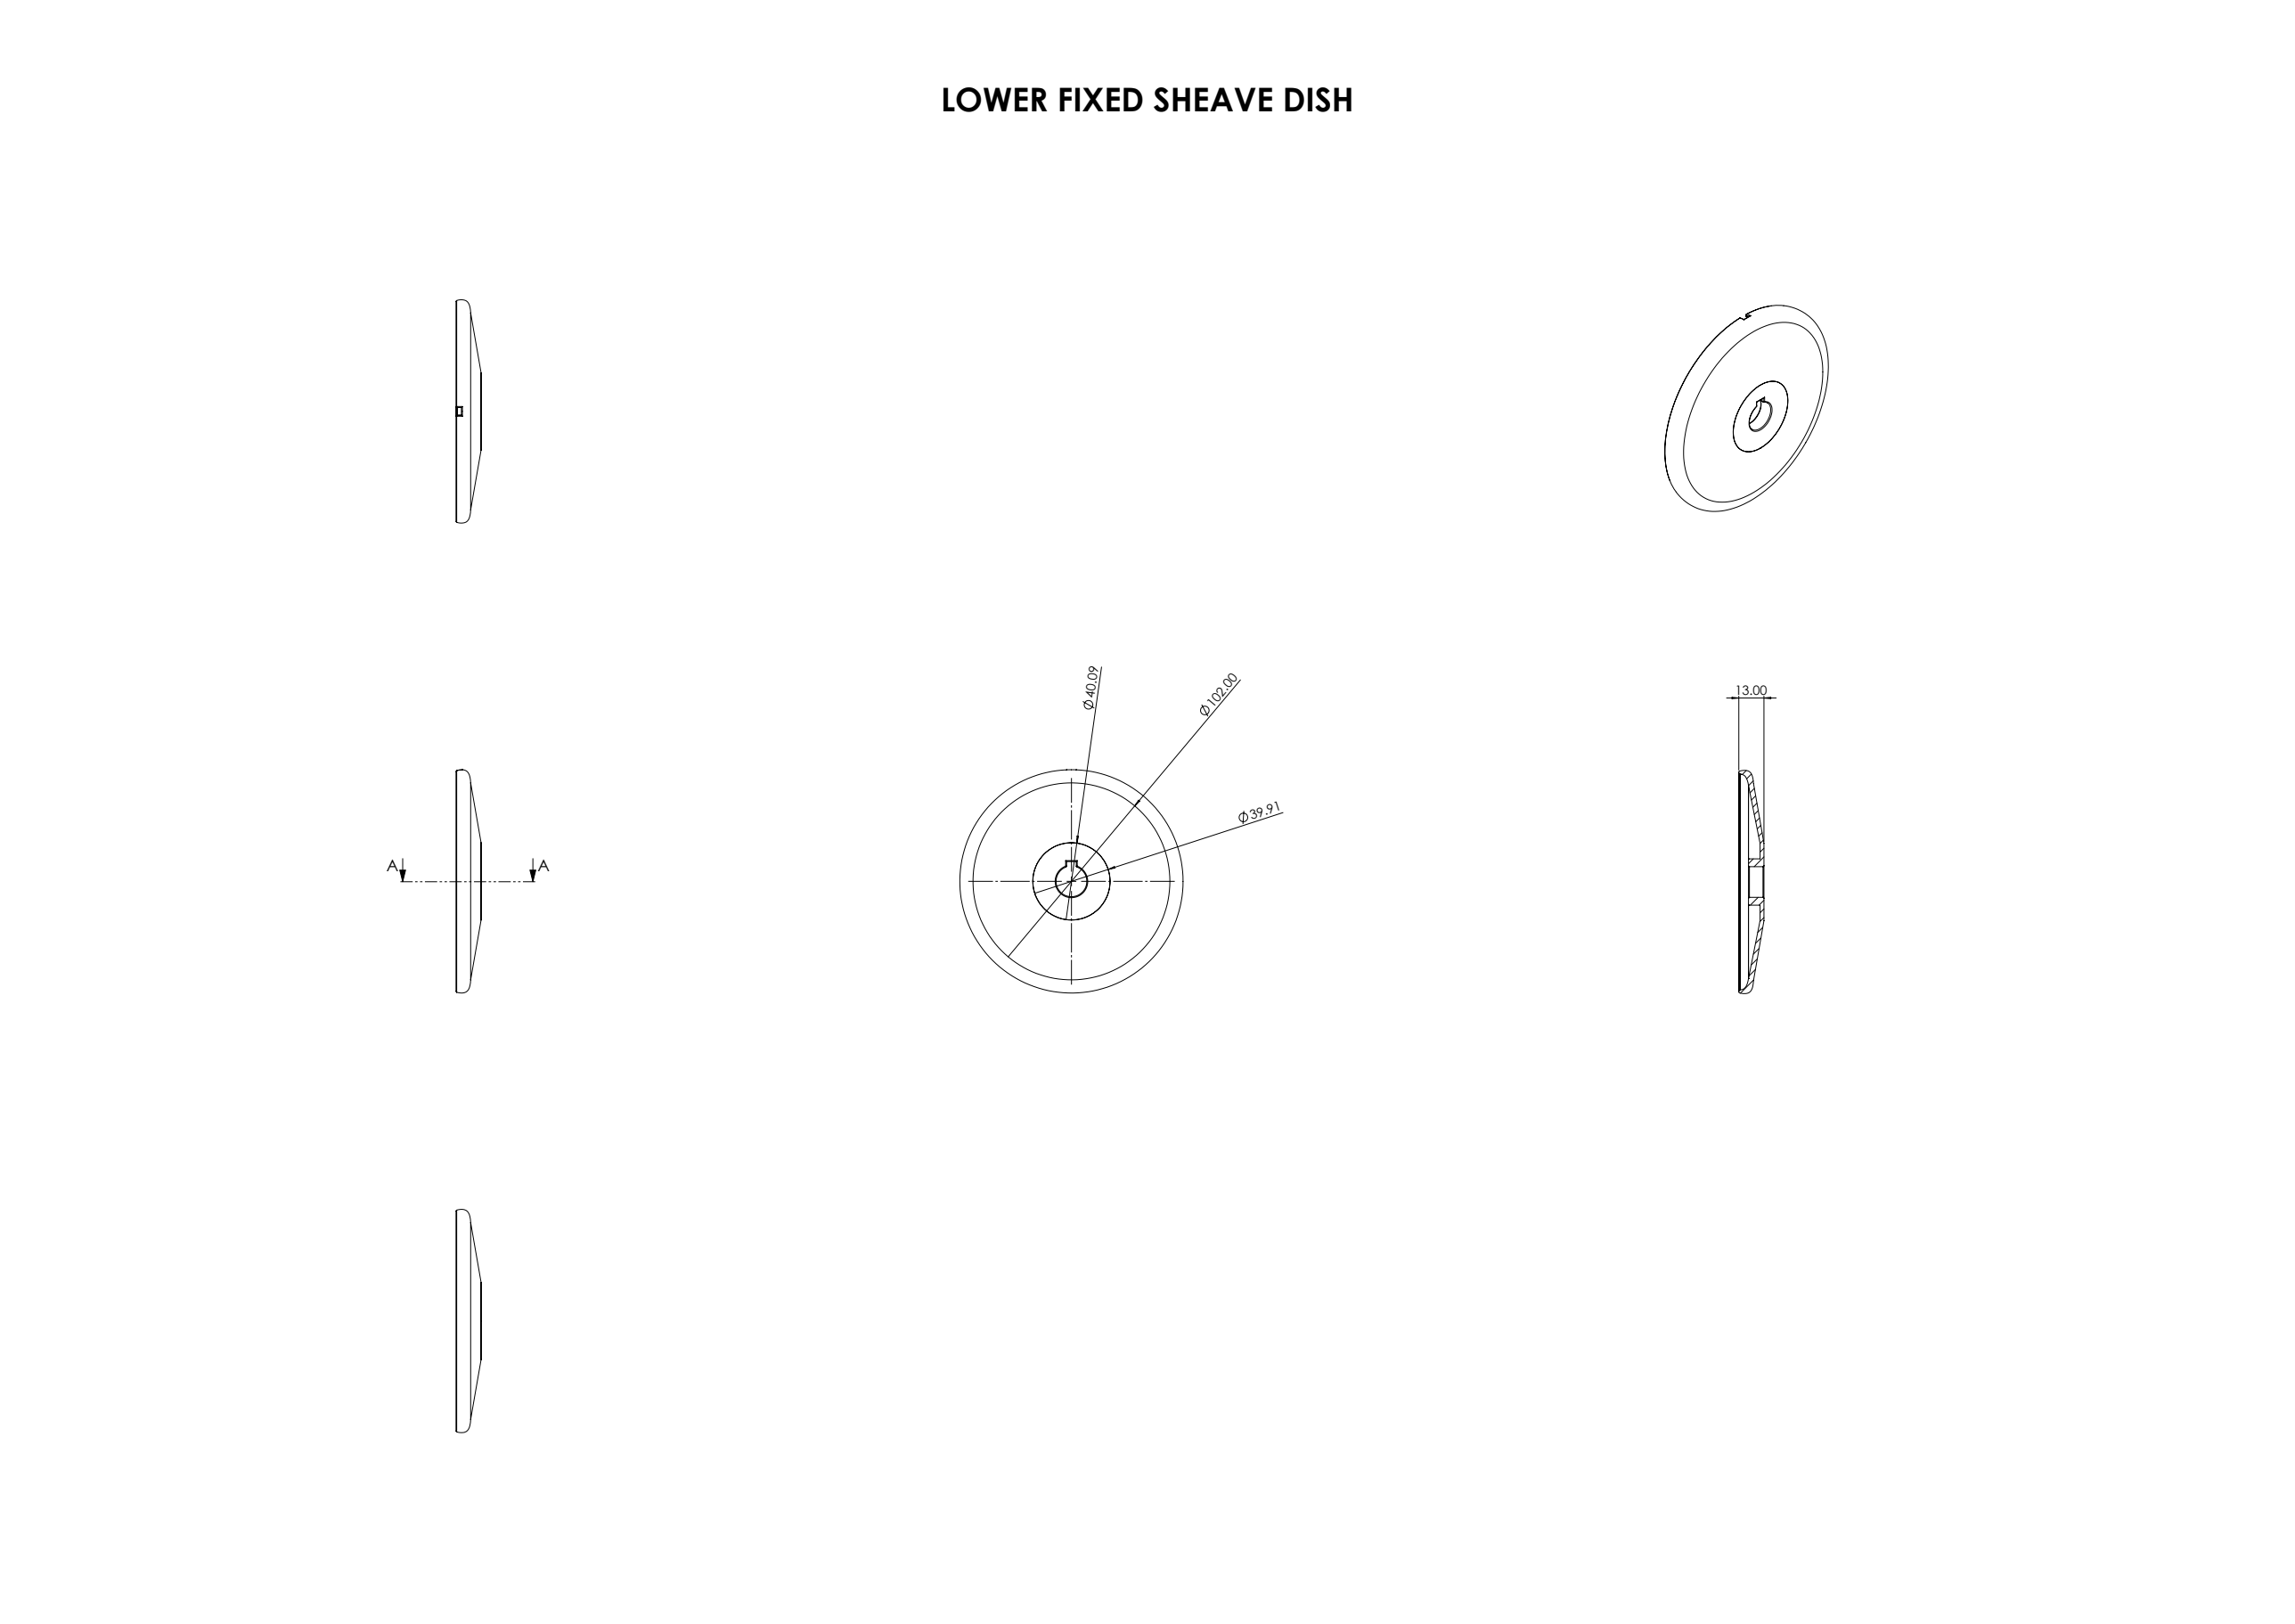
ISO-10303-21;
HEADER;
/* Generated by software containing ST-Developer
 * from STEP Tools, Inc. (www.steptools.com) 
 */

FILE_DESCRIPTION(
/* description */ (''),
/* implementation_level */ '2;1');

FILE_NAME(
/* name */ '04_Lower_Fixed_Sheave_Dish.step',
/* time_stamp */ '2026-10-24T13:41:11-07:00',
/* author */ (''),
/* organization */ (''),
/* preprocessor_version */ 'ST-DEVELOPER v20.2',
/* originating_system */ 'Autodesk Translation Framework v15.15.0.0',
/* authorisation */ '');

FILE_SCHEMA (('AUTOMOTIVE_DESIGN { 1 0 10303 214 3 1 1 }'));
ENDSEC;

DATA;
#10=MECHANICAL_DESIGN_GEOMETRIC_PRESENTATION_REPRESENTATION('',(#124),#12813);
#63=ELLIPSE('',#4739,0.707106781186547,0.5);
#64=ELLIPSE('',#4740,0.707106781186547,0.5);
#65=ELLIPSE('',#4754,0.707106781186549,0.5);
#66=ELLIPSE('',#4755,0.707106781186547,0.5);
#67=SPHERICAL_SURFACE('',#4710,0.5);
#68=SPHERICAL_SURFACE('',#4712,0.5);
#69=SPHERICAL_SURFACE('',#4720,0.5);
#70=SPHERICAL_SURFACE('',#4723,0.5);
#71=SPHERICAL_SURFACE('',#4743,0.5);
#72=SPHERICAL_SURFACE('',#4756,0.5);
#73=SPHERICAL_SURFACE('',#4773,0.5);
#74=SPHERICAL_SURFACE('',#4779,0.5);
#75=SPHERICAL_SURFACE('',#4788,0.5);
#76=SPHERICAL_SURFACE('',#4790,0.5);
#89=CONICAL_SURFACE('',#4727,35.,1.37340076694502);
#90=CONICAL_SURFACE('',#4770,35.5,1.39833325526807);
#91=CONICAL_SURFACE('',#4795,56.05,0.694738276196701);
#104=SHAPE_REPRESENTATION_RELATIONSHIP('SRR','None',#12857,#114);
#114=ADVANCED_BREP_SHAPE_REPRESENTATION('',(#134),#12806);
#124=STYLED_ITEM('',(#12967),#134);
#134=MANIFOLD_SOLID_BREP('Body1',#4387);
#153=FACE_BOUND('',#738,.T.);
#154=FACE_BOUND('',#753,.T.);
#155=FACE_BOUND('',#774,.T.);
#196=PLANE('',#4717);
#197=PLANE('',#4725);
#198=PLANE('',#4734);
#199=PLANE('',#4751);
#200=PLANE('',#4752);
#201=PLANE('',#4769);
#202=PLANE('',#4781);
#203=PLANE('',#4792);
#204=PLANE('',#4793);
#205=PLANE('',#4794);
#272=TOROIDAL_SURFACE('',#4705,56.5341874729922,0.5);
#273=TOROIDAL_SURFACE('',#4729,11.5,0.5);
#274=TOROIDAL_SURFACE('',#4746,8.45,0.5);
#275=TOROIDAL_SURFACE('',#4760,8.45,0.5);
#276=TOROIDAL_SURFACE('',#4764,19.9567770454363,0.5);
#292=(
BOUNDED_CURVE()
B_SPLINE_CURVE(5,(#10926,#10927,#10928,#10929,#10930,#10931,#10932,#10933,
#10934,#10935,#10936,#10937,#10938,#10939,#10940),.UNSPECIFIED.,.F.,.F.)
B_SPLINE_CURVE_WITH_KNOTS((6,1,1,1,1,1,1,1,1,1,6),(0.000900413620571326,
0.0666666666666667,0.133333333333333,0.2,0.266666666666667,0.333333333333333,
0.4,0.466666666666667,0.533333333333333,0.6,0.62572757688512),
 .UNSPECIFIED.)
CURVE()
GEOMETRIC_REPRESENTATION_ITEM()
RATIONAL_B_SPLINE_CURVE((1.,1.,1.,1.,1.,1.,1.,1.,1.,1.,1.,1.,1.,1.,1.))
REPRESENTATION_ITEM('')
);
#293=(
BOUNDED_CURVE()
B_SPLINE_CURVE(5,(#11656,#11657,#11658,#11659,#11660,#11661,#11662,#11663,
#11664,#11665,#11666,#11667,#11668,#11669,#11670,#11671,#11672,#11673,#11674),
 .UNSPECIFIED.,.F.,.F.)
B_SPLINE_CURVE_WITH_KNOTS((6,1,1,1,1,1,1,1,1,1,1,1,1,1,6),(0.323025444096601,
0.35,0.4,0.45,0.5,0.55,0.6,0.65,0.7,0.75,0.8,0.85,0.9,0.95,1.),
 .UNSPECIFIED.)
CURVE()
GEOMETRIC_REPRESENTATION_ITEM()
RATIONAL_B_SPLINE_CURVE((1.,1.,1.,1.,1.,1.,1.,1.,1.,1.,1.,1.,1.,1.,1.,1.,
1.,1.,1.))
REPRESENTATION_ITEM('')
);
#296=(
BOUNDED_SURFACE()
B_SPLINE_SURFACE(5,2,((#10735,#10736,#10737,#10738,#10739,#10740,#10741,
#10742,#10743),(#10744,#10745,#10746,#10747,#10748,#10749,#10750,#10751,
#10752),(#10753,#10754,#10755,#10756,#10757,#10758,#10759,#10760,#10761),
(#10762,#10763,#10764,#10765,#10766,#10767,#10768,#10769,#10770),(#10771,
#10772,#10773,#10774,#10775,#10776,#10777,#10778,#10779),(#10780,#10781,
#10782,#10783,#10784,#10785,#10786,#10787,#10788),(#10789,#10790,#10791,
#10792,#10793,#10794,#10795,#10796,#10797),(#10798,#10799,#10800,#10801,
#10802,#10803,#10804,#10805,#10806),(#10807,#10808,#10809,#10810,#10811,
#10812,#10813,#10814,#10815),(#10816,#10817,#10818,#10819,#10820,#10821,
#10822,#10823,#10824),(#10825,#10826,#10827,#10828,#10829,#10830,#10831,
#10832,#10833),(#10834,#10835,#10836,#10837,#10838,#10839,#10840,#10841,
#10842),(#10843,#10844,#10845,#10846,#10847,#10848,#10849,#10850,#10851),
(#10852,#10853,#10854,#10855,#10856,#10857,#10858,#10859,#10860),(#10861,
#10862,#10863,#10864,#10865,#10866,#10867,#10868,#10869),(#10870,#10871,
#10872,#10873,#10874,#10875,#10876,#10877,#10878),(#10879,#10880,#10881,
#10882,#10883,#10884,#10885,#10886,#10887),(#10888,#10889,#10890,#10891,
#10892,#10893,#10894,#10895,#10896),(#10897,#10898,#10899,#10900,#10901,
#10902,#10903,#10904,#10905),(#10906,#10907,#10908,#10909,#10910,#10911,
#10912,#10913,#10914)),.UNSPECIFIED.,.F.,.T.,.F.)
B_SPLINE_SURFACE_WITH_KNOTS((6,1,1,1,1,1,1,1,1,1,1,1,1,1,1,6),(3,2,2,2,
3),(-1.,-0.933333333333333,-0.866666666666667,-0.8,-0.733333333333333,-0.666666666666667,
-0.6,-0.533333333333333,-0.466666666666667,-0.4,-0.333333333333333,-0.266666666666667,
-0.2,-0.133333333333333,-0.0666666666666667,0.),(0.,1.5707963267949,3.14159265358979,
4.71238898038469,6.28318530717959),.UNSPECIFIED.)
GEOMETRIC_REPRESENTATION_ITEM()
RATIONAL_B_SPLINE_SURFACE(((1.,0.707106781186548,1.,0.707106781186548,1.,
0.707106781186548,1.,0.707106781186548,1.),(1.,0.707106781186548,1.,0.707106781186548,
1.,0.707106781186548,1.,0.707106781186548,1.),(1.,0.707106781186548,1.,
0.707106781186548,1.,0.707106781186548,1.,0.707106781186548,1.),(1.,0.707106781186548,
1.,0.707106781186548,1.,0.707106781186548,1.,0.707106781186548,1.),(1.,
0.707106781186548,1.,0.707106781186548,1.,0.707106781186548,1.,0.707106781186548,
1.),(1.,0.707106781186548,1.,0.707106781186548,1.,0.707106781186548,1.,
0.707106781186548,1.),(1.,0.707106781186548,1.,0.707106781186548,1.,0.707106781186548,
1.,0.707106781186548,1.),(1.,0.707106781186548,1.,0.707106781186548,1.,
0.707106781186548,1.,0.707106781186548,1.),(1.,0.707106781186548,1.,0.707106781186548,
1.,0.707106781186548,1.,0.707106781186548,1.),(1.,0.707106781186548,1.,
0.707106781186548,1.,0.707106781186548,1.,0.707106781186548,1.),(1.,0.707106781186548,
1.,0.707106781186548,1.,0.707106781186548,1.,0.707106781186548,1.),(1.,
0.707106781186548,1.,0.707106781186548,1.,0.707106781186548,1.,0.707106781186548,
1.),(1.,0.707106781186548,1.,0.707106781186548,1.,0.707106781186548,1.,
0.707106781186548,1.),(1.,0.707106781186548,1.,0.707106781186548,1.,0.707106781186548,
1.,0.707106781186548,1.),(1.,0.707106781186548,1.,0.707106781186548,1.,
0.707106781186548,1.,0.707106781186548,1.),(1.,0.707106781186548,1.,0.707106781186548,
1.,0.707106781186548,1.,0.707106781186548,1.),(1.,0.707106781186548,1.,
0.707106781186548,1.,0.707106781186548,1.,0.707106781186548,1.),(1.,0.707106781186548,
1.,0.707106781186548,1.,0.707106781186548,1.,0.707106781186548,1.),(1.,
0.707106781186548,1.,0.707106781186548,1.,0.707106781186548,1.,0.707106781186548,
1.),(1.,0.707106781186548,1.,0.707106781186548,1.,0.707106781186548,1.,
0.707106781186548,1.)))
REPRESENTATION_ITEM('')
SURFACE()
);
#297=(
BOUNDED_SURFACE()
B_SPLINE_SURFACE(5,2,((#11421,#11422,#11423,#11424,#11425,#11426,#11427,
#11428,#11429),(#11430,#11431,#11432,#11433,#11434,#11435,#11436,#11437,
#11438),(#11439,#11440,#11441,#11442,#11443,#11444,#11445,#11446,#11447),
(#11448,#11449,#11450,#11451,#11452,#11453,#11454,#11455,#11456),(#11457,
#11458,#11459,#11460,#11461,#11462,#11463,#11464,#11465),(#11466,#11467,
#11468,#11469,#11470,#11471,#11472,#11473,#11474),(#11475,#11476,#11477,
#11478,#11479,#11480,#11481,#11482,#11483),(#11484,#11485,#11486,#11487,
#11488,#11489,#11490,#11491,#11492),(#11493,#11494,#11495,#11496,#11497,
#11498,#11499,#11500,#11501),(#11502,#11503,#11504,#11505,#11506,#11507,
#11508,#11509,#11510),(#11511,#11512,#11513,#11514,#11515,#11516,#11517,
#11518,#11519),(#11520,#11521,#11522,#11523,#11524,#11525,#11526,#11527,
#11528),(#11529,#11530,#11531,#11532,#11533,#11534,#11535,#11536,#11537),
(#11538,#11539,#11540,#11541,#11542,#11543,#11544,#11545,#11546),(#11547,
#11548,#11549,#11550,#11551,#11552,#11553,#11554,#11555),(#11556,#11557,
#11558,#11559,#11560,#11561,#11562,#11563,#11564),(#11565,#11566,#11567,
#11568,#11569,#11570,#11571,#11572,#11573),(#11574,#11575,#11576,#11577,
#11578,#11579,#11580,#11581,#11582),(#11583,#11584,#11585,#11586,#11587,
#11588,#11589,#11590,#11591),(#11592,#11593,#11594,#11595,#11596,#11597,
#11598,#11599,#11600),(#11601,#11602,#11603,#11604,#11605,#11606,#11607,
#11608,#11609),(#11610,#11611,#11612,#11613,#11614,#11615,#11616,#11617,
#11618),(#11619,#11620,#11621,#11622,#11623,#11624,#11625,#11626,#11627),
(#11628,#11629,#11630,#11631,#11632,#11633,#11634,#11635,#11636),(#11637,
#11638,#11639,#11640,#11641,#11642,#11643,#11644,#11645)),.UNSPECIFIED.,
 .F.,.T.,.F.)
B_SPLINE_SURFACE_WITH_KNOTS((6,1,1,1,1,1,1,1,1,1,1,1,1,1,1,1,1,1,1,1,6),
(3,2,2,2,3),(-1.,-0.95,-0.9,-0.85,-0.8,-0.75,-0.7,-0.65,-0.6,-0.55,-0.5,
-0.45,-0.4,-0.35,-0.3,-0.25,-0.2,-0.15,-0.1,-0.05,0.),(0.,1.5707963267949,
3.14159265358979,4.71238898038469,6.28318530717959),.UNSPECIFIED.)
GEOMETRIC_REPRESENTATION_ITEM()
RATIONAL_B_SPLINE_SURFACE(((1.,0.707106781186548,1.,0.707106781186548,1.,
0.707106781186548,1.,0.707106781186548,1.),(1.,0.707106781186548,1.,0.707106781186548,
1.,0.707106781186548,1.,0.707106781186548,1.),(1.,0.707106781186548,1.,
0.707106781186548,1.,0.707106781186548,1.,0.707106781186548,1.),(1.,0.707106781186548,
1.,0.707106781186548,1.,0.707106781186548,1.,0.707106781186548,1.),(1.,
0.707106781186548,1.,0.707106781186548,1.,0.707106781186548,1.,0.707106781186548,
1.),(1.,0.707106781186548,1.,0.707106781186548,1.,0.707106781186548,1.,
0.707106781186548,1.),(1.,0.707106781186548,1.,0.707106781186548,1.,0.707106781186548,
1.,0.707106781186548,1.),(1.,0.707106781186548,1.,0.707106781186548,1.,
0.707106781186548,1.,0.707106781186548,1.),(1.,0.707106781186548,1.,0.707106781186548,
1.,0.707106781186548,1.,0.707106781186548,1.),(1.,0.707106781186548,1.,
0.707106781186548,1.,0.707106781186548,1.,0.707106781186548,1.),(1.,0.707106781186548,
1.,0.707106781186548,1.,0.707106781186548,1.,0.707106781186548,1.),(1.,
0.707106781186548,1.,0.707106781186548,1.,0.707106781186548,1.,0.707106781186548,
1.),(1.,0.707106781186548,1.,0.707106781186548,1.,0.707106781186548,1.,
0.707106781186548,1.),(1.,0.707106781186548,1.,0.707106781186548,1.,0.707106781186548,
1.,0.707106781186548,1.),(1.,0.707106781186548,1.,0.707106781186548,1.,
0.707106781186548,1.,0.707106781186548,1.),(1.,0.707106781186548,1.,0.707106781186548,
1.,0.707106781186548,1.,0.707106781186548,1.),(1.,0.707106781186548,1.,
0.707106781186548,1.,0.707106781186548,1.,0.707106781186548,1.),(1.,0.707106781186548,
1.,0.707106781186548,1.,0.707106781186548,1.,0.707106781186548,1.),(1.,
0.707106781186548,1.,0.707106781186548,1.,0.707106781186548,1.,0.707106781186548,
1.),(1.,0.707106781186548,1.,0.707106781186548,1.,0.707106781186548,1.,
0.707106781186548,1.),(1.,0.707106781186548,1.,0.707106781186548,1.,0.707106781186548,
1.,0.707106781186548,1.),(1.,0.707106781186548,1.,0.707106781186548,1.,
0.707106781186548,1.,0.707106781186548,1.),(1.,0.707106781186548,1.,0.707106781186548,
1.,0.707106781186548,1.,0.707106781186548,1.),(1.,0.707106781186548,1.,
0.707106781186548,1.,0.707106781186548,1.,0.707106781186548,1.),(1.,0.707106781186548,
1.,0.707106781186548,1.,0.707106781186548,1.,0.707106781186548,1.)))
REPRESENTATION_ITEM('')
SURFACE()
);
#308=B_SPLINE_SURFACE_WITH_KNOTS('',3,3,((#10445,#10446,#10447,#10448),
(#10449,#10450,#10451,#10452),(#10453,#10454,#10455,#10456),(#10457,#10458,
#10459,#10460),(#10461,#10462,#10463,#10464)),.UNSPECIFIED.,.F.,.F.,.F.,
(4,1,4),(4,4),(0.,0.5,1.),(0.088693979487329,0.125274232772668),
 .UNSPECIFIED.);
#309=B_SPLINE_SURFACE_WITH_KNOTS('',3,3,((#10506,#10507,#10508,#10509,#10510,
#10511,#10512,#10513,#10514,#10515,#10516,#10517,#10518,#10519,#10520,#10521,
#10522,#10523,#10524,#10525,#10526,#10527),(#10528,#10529,#10530,#10531,
#10532,#10533,#10534,#10535,#10536,#10537,#10538,#10539,#10540,#10541,#10542,
#10543,#10544,#10545,#10546,#10547,#10548,#10549),(#10550,#10551,#10552,
#10553,#10554,#10555,#10556,#10557,#10558,#10559,#10560,#10561,#10562,#10563,
#10564,#10565,#10566,#10567,#10568,#10569,#10570,#10571),(#10572,#10573,
#10574,#10575,#10576,#10577,#10578,#10579,#10580,#10581,#10582,#10583,#10584,
#10585,#10586,#10587,#10588,#10589,#10590,#10591,#10592,#10593)),
 .UNSPECIFIED.,.F.,.F.,.F.,(4,4),(4,1,1,1,1,1,1,1,1,1,1,1,1,1,1,1,1,1,1,
4),(0.,1.),(0.,2.49089996579439,4.98179993158877,6.64239990878503,8.30299988598129,
9.96359986317755,11.6241998403738,13.2847998175701,14.9453997947663,16.6059997719626,
18.2665997491588,19.9271997263551,21.5877997035514,23.2483996807476,24.9089996579439,
26.5695996351401,28.2301996123364,29.8907995895326,32.381699555327,34.8725995211214),
 .UNSPECIFIED.);
#310=B_SPLINE_SURFACE_WITH_KNOTS('',3,3,((#10649,#10650,#10651,#10652),
(#10653,#10654,#10655,#10656),(#10657,#10658,#10659,#10660),(#10661,#10662,
#10663,#10664),(#10665,#10666,#10667,#10668)),.UNSPECIFIED.,.F.,.F.,.F.,
(4,1,4),(4,4),(0.,0.5,1.),(0.0886939794873267,0.125274232772633),
 .UNSPECIFIED.);
#311=B_SPLINE_SURFACE_WITH_KNOTS('',3,3,((#10677,#10678,#10679,#10680),
(#10681,#10682,#10683,#10684),(#10685,#10686,#10687,#10688),(#10689,#10690,
#10691,#10692)),.UNSPECIFIED.,.F.,.F.,.F.,(4,4),(4,4),(0.,1.),(0.587131769179142,
0.860462555942468),.UNSPECIFIED.);
#312=B_SPLINE_SURFACE_WITH_KNOTS('',3,3,((#10968,#10969,#10970,#10971),
(#10972,#10973,#10974,#10975),(#10976,#10977,#10978,#10979),(#10980,#10981,
#10982,#10983)),.UNSPECIFIED.,.F.,.F.,.F.,(4,4),(4,4),(0.,1.),(0.0190073922957582,
0.292336438831091),.UNSPECIFIED.);
#313=B_SPLINE_SURFACE_WITH_KNOTS('',3,3,((#11013,#11014,#11015,#11016,#11017,
#11018,#11019,#11020,#11021,#11022,#11023,#11024,#11025,#11026,#11027,#11028,
#11029,#11030,#11031,#11032,#11033,#11034,#11035),(#11036,#11037,#11038,
#11039,#11040,#11041,#11042,#11043,#11044,#11045,#11046,#11047,#11048,#11049,
#11050,#11051,#11052,#11053,#11054,#11055,#11056,#11057,#11058),(#11059,
#11060,#11061,#11062,#11063,#11064,#11065,#11066,#11067,#11068,#11069,#11070,
#11071,#11072,#11073,#11074,#11075,#11076,#11077,#11078,#11079,#11080,#11081),
(#11082,#11083,#11084,#11085,#11086,#11087,#11088,#11089,#11090,#11091,
#11092,#11093,#11094,#11095,#11096,#11097,#11098,#11099,#11100,#11101,#11102,
#11103,#11104)),.UNSPECIFIED.,.F.,.T.,.F.,(4,4),(4,1,1,1,1,1,1,1,1,1,1,
1,1,1,1,1,1,1,1,1,4),(0.,1.),(1.5707963267949,2.01959527730772,2.46839422782055,
2.76759352816244,3.06679282850432,3.36599212884621,3.66519142918809,3.96439072952998,
4.26359002987186,4.56278933021375,4.86198863055563,5.16118793089752,5.4603872312394,
5.75958653158129,6.05878583192317,6.20838548209412,6.35798513226506,6.65718443260694,
6.95638373294883,7.40518268346166,7.85398163397448),.UNSPECIFIED.);
#314=B_SPLINE_SURFACE_WITH_KNOTS('',3,3,((#11243,#11244,#11245,#11246,#11247,
#11248,#11249,#11250,#11251,#11252,#11253,#11254,#11255,#11256,#11257,#11258,
#11259,#11260,#11261,#11262,#11263),(#11264,#11265,#11266,#11267,#11268,
#11269,#11270,#11271,#11272,#11273,#11274,#11275,#11276,#11277,#11278,#11279,
#11280,#11281,#11282,#11283,#11284),(#11285,#11286,#11287,#11288,#11289,
#11290,#11291,#11292,#11293,#11294,#11295,#11296,#11297,#11298,#11299,#11300,
#11301,#11302,#11303,#11304,#11305),(#11306,#11307,#11308,#11309,#11310,
#11311,#11312,#11313,#11314,#11315,#11316,#11317,#11318,#11319,#11320,#11321,
#11322,#11323,#11324,#11325,#11326),(#11327,#11328,#11329,#11330,#11331,
#11332,#11333,#11334,#11335,#11336,#11337,#11338,#11339,#11340,#11341,#11342,
#11343,#11344,#11345,#11346,#11347)),.UNSPECIFIED.,.F.,.F.,.F.,(4,1,4),
(4,1,1,1,1,1,1,1,1,1,1,1,1,1,1,1,1,1,4),(0.,0.5,1.),(0.,2.5201892997592,
5.0403785995184,6.72050479935786,8.40063099919733,10.0807571990368,11.7608833988763,
15.1211357985552,15.9611988984749,16.8012619983947,20.1615143980736,21.841640597913,
23.5217667977525,25.201892997592,26.8820191974314,28.5621453972709,30.2422715971104,
32.7624608968696,35.2826501966288),.UNSPECIFIED.);
#315=B_SPLINE_SURFACE_WITH_KNOTS('',3,3,((#11381,#11382,#11383,#11384),
(#11385,#11386,#11387,#11388),(#11389,#11390,#11391,#11392),(#11393,#11394,
#11395,#11396)),.UNSPECIFIED.,.F.,.F.,.F.,(4,4),(4,4),(0.,1.),(0.825569897711632,
1.1096475233552),.UNSPECIFIED.);
#316=B_SPLINE_SURFACE_WITH_KNOTS('',3,3,((#11679,#11680,#11681,#11682),
(#11683,#11684,#11685,#11686),(#11687,#11688,#11689,#11690),(#11691,#11692,
#11693,#11694)),.UNSPECIFIED.,.F.,.F.,.F.,(4,4),(4,4),(0.,1.),(0.0332835073847237,
0.317361133028268),.UNSPECIFIED.);
#317=B_SPLINE_SURFACE_WITH_KNOTS('',3,3,((#11721,#11722,#11723,#11724),
(#11725,#11726,#11727,#11728),(#11729,#11730,#11731,#11732),(#11733,#11734,
#11735,#11736)),.UNSPECIFIED.,.F.,.F.,.F.,(4,4),(4,4),(0.,1.),(34.6574150541607,
35.1575805274809),.UNSPECIFIED.);
#318=B_SPLINE_SURFACE_WITH_KNOTS('',3,3,((#11766,#11767,#11768,#11769),
(#11770,#11771,#11772,#11773),(#11774,#11775,#11776,#11777),(#11778,#11779,
#11780,#11781),(#11782,#11783,#11784,#11785)),.UNSPECIFIED.,.F.,.F.,.F.,
(4,1,4),(4,4),(0.,0.5,1.),(35.8573857487427,36.3575403182),
 .UNSPECIFIED.);
#438=FACE_OUTER_BOUND('',#720,.T.);
#439=FACE_OUTER_BOUND('',#721,.T.);
#440=FACE_OUTER_BOUND('',#722,.T.);
#441=FACE_OUTER_BOUND('',#723,.T.);
#442=FACE_OUTER_BOUND('',#724,.T.);
#443=FACE_OUTER_BOUND('',#725,.T.);
#444=FACE_OUTER_BOUND('',#726,.T.);
#445=FACE_OUTER_BOUND('',#727,.T.);
#446=FACE_OUTER_BOUND('',#728,.T.);
#447=FACE_OUTER_BOUND('',#729,.T.);
#448=FACE_OUTER_BOUND('',#730,.T.);
#449=FACE_OUTER_BOUND('',#731,.T.);
#450=FACE_OUTER_BOUND('',#732,.T.);
#451=FACE_OUTER_BOUND('',#733,.T.);
#452=FACE_OUTER_BOUND('',#734,.T.);
#453=FACE_OUTER_BOUND('',#735,.T.);
#454=FACE_OUTER_BOUND('',#736,.T.);
#455=FACE_OUTER_BOUND('',#737,.T.);
#456=FACE_OUTER_BOUND('',#739,.T.);
#457=FACE_OUTER_BOUND('',#740,.T.);
#458=FACE_OUTER_BOUND('',#741,.T.);
#459=FACE_OUTER_BOUND('',#742,.T.);
#460=FACE_OUTER_BOUND('',#743,.T.);
#461=FACE_OUTER_BOUND('',#744,.T.);
#462=FACE_OUTER_BOUND('',#745,.T.);
#463=FACE_OUTER_BOUND('',#746,.T.);
#464=FACE_OUTER_BOUND('',#747,.T.);
#465=FACE_OUTER_BOUND('',#748,.T.);
#466=FACE_OUTER_BOUND('',#749,.T.);
#467=FACE_OUTER_BOUND('',#750,.T.);
#468=FACE_OUTER_BOUND('',#751,.T.);
#469=FACE_OUTER_BOUND('',#752,.T.);
#470=FACE_OUTER_BOUND('',#754,.T.);
#471=FACE_OUTER_BOUND('',#755,.T.);
#472=FACE_OUTER_BOUND('',#756,.T.);
#473=FACE_OUTER_BOUND('',#757,.T.);
#474=FACE_OUTER_BOUND('',#758,.T.);
#475=FACE_OUTER_BOUND('',#759,.T.);
#476=FACE_OUTER_BOUND('',#760,.T.);
#477=FACE_OUTER_BOUND('',#761,.T.);
#478=FACE_OUTER_BOUND('',#762,.T.);
#479=FACE_OUTER_BOUND('',#763,.T.);
#480=FACE_OUTER_BOUND('',#764,.T.);
#481=FACE_OUTER_BOUND('',#765,.T.);
#482=FACE_OUTER_BOUND('',#766,.T.);
#483=FACE_OUTER_BOUND('',#767,.T.);
#484=FACE_OUTER_BOUND('',#768,.T.);
#485=FACE_OUTER_BOUND('',#769,.T.);
#486=FACE_OUTER_BOUND('',#770,.T.);
#487=FACE_OUTER_BOUND('',#771,.T.);
#488=FACE_OUTER_BOUND('',#772,.T.);
#489=FACE_OUTER_BOUND('',#773,.T.);
#490=FACE_OUTER_BOUND('',#775,.T.);
#720=EDGE_LOOP('',(#3331,#3332,#3333,#3334));
#721=EDGE_LOOP('',(#3335,#3336,#3337));
#722=EDGE_LOOP('',(#3338,#3339,#3340));
#723=EDGE_LOOP('',(#3341,#3342,#3343,#3344));
#724=EDGE_LOOP('',(#3345,#3346,#3347,#3348));
#725=EDGE_LOOP('',(#3349,#3350,#3351,#3352));
#726=EDGE_LOOP('',(#3353,#3354,#3355,#3356));
#727=EDGE_LOOP('',(#3357,#3358,#3359));
#728=EDGE_LOOP('',(#3360,#3361,#3362));
#729=EDGE_LOOP('',(#3363,#3364,#3365,#3366));
#730=EDGE_LOOP('',(#3367,#3368,#3369,#3370,#3371));
#731=EDGE_LOOP('',(#3372,#3373,#3374,#3375,#3376,#3377,#3378,#3379));
#732=EDGE_LOOP('',(#3380,#3381,#3382,#3383,#3384));
#733=EDGE_LOOP('',(#3385,#3386,#3387,#3388,#3389));
#734=EDGE_LOOP('',(#3390,#3391,#3392,#3393,#3394));
#735=EDGE_LOOP('',(#3395,#3396,#3397,#3398,#3399));
#736=EDGE_LOOP('',(#3400,#3401,#3402,#3403,#3404));
#737=EDGE_LOOP('',(#3405));
#738=EDGE_LOOP('',(#3406,#3407,#3408,#3409));
#739=EDGE_LOOP('',(#3410,#3411,#3412,#3413,#3414));
#740=EDGE_LOOP('',(#3415,#3416,#3417,#3418));
#741=EDGE_LOOP('',(#3419,#3420,#3421,#3422));
#742=EDGE_LOOP('',(#3423,#3424,#3425));
#743=EDGE_LOOP('',(#3426,#3427,#3428,#3429));
#744=EDGE_LOOP('',(#3430,#3431,#3432,#3433));
#745=EDGE_LOOP('',(#3434,#3435,#3436,#3437));
#746=EDGE_LOOP('',(#3438,#3439,#3440,#3441));
#747=EDGE_LOOP('',(#3442,#3443,#3444,#3445));
#748=EDGE_LOOP('',(#3446,#3447,#3448));
#749=EDGE_LOOP('',(#3449,#3450,#3451,#3452));
#750=EDGE_LOOP('',(#3453,#3454,#3455,#3456));
#751=EDGE_LOOP('',(#3457,#3458,#3459,#3460,#3461));
#752=EDGE_LOOP('',(#3462));
#753=EDGE_LOOP('',(#3463,#3464,#3465,#3466));
#754=EDGE_LOOP('',(#3467,#3468,#3469,#3470,#3471,#3472));
#755=EDGE_LOOP('',(#3473,#3474,#3475));
#756=EDGE_LOOP('',(#3476,#3477,#3478,#3479));
#757=EDGE_LOOP('',(#3480,#3481,#3482,#3483));
#758=EDGE_LOOP('',(#3484,#3485,#3486));
#759=EDGE_LOOP('',(#3487,#3488,#3489,#3490));
#760=EDGE_LOOP('',(#3491,#3492,#3493,#3494));
#761=EDGE_LOOP('',(#3495,#3496,#3497,#3498));
#762=EDGE_LOOP('',(#3499,#3500,#3501,#3502));
#763=EDGE_LOOP('',(#3503,#3504,#3505,#3506));
#764=EDGE_LOOP('',(#3507,#3508,#3509));
#765=EDGE_LOOP('',(#3510,#3511,#3512));
#766=EDGE_LOOP('',(#3513,#3514,#3515,#3516,#3517));
#767=EDGE_LOOP('',(#3518,#3519,#3520,#3521,#3522,#3523,#3524,#3525,#3526));
#768=EDGE_LOOP('',(#3527,#3528,#3529,#3530,#3531));
#769=EDGE_LOOP('',(#3532,#3533,#3534,#3535,#3536));
#770=EDGE_LOOP('',(#3537,#3538,#3539,#3540,#3541,#3542,#3543));
#771=EDGE_LOOP('',(#3544,#3545,#3546,#3547,#3548,#3549,#3550,#3551,#3552,
#3553,#3554,#3555));
#772=EDGE_LOOP('',(#3556,#3557,#3558,#3559,#3560,#3561,#3562));
#773=EDGE_LOOP('',(#3563));
#774=EDGE_LOOP('',(#3564));
#775=EDGE_LOOP('',(#3565,#3566,#3567,#3568));
#985=CIRCLE('',#4706,0.5);
#986=CIRCLE('',#4707,56.1500768331935);
#987=CIRCLE('',#4708,0.499999999998982);
#988=CIRCLE('',#4709,56.5341874729922);
#989=CIRCLE('',#4711,0.5);
#990=CIRCLE('',#4713,0.5);
#991=CIRCLE('',#4714,0.50000000000007);
#992=CIRCLE('',#4716,0.5);
#993=CIRCLE('',#4718,0.499999999999984);
#994=CIRCLE('',#4719,0.499999999999998);
#995=CIRCLE('',#4721,0.499999999999986);
#996=CIRCLE('',#4722,0.499999999999986);
#997=CIRCLE('',#4724,0.5);
#998=CIRCLE('',#4726,0.500000000000001);
#999=CIRCLE('',#4728,20.);
#1000=CIRCLE('',#4730,12.);
#1001=CIRCLE('',#4731,12.);
#1002=CIRCLE('',#4732,0.5);
#1003=CIRCLE('',#4733,11.5);
#1004=CIRCLE('',#4735,8.45);
#1005=CIRCLE('',#4737,12.);
#1006=CIRCLE('',#4742,0.5);
#1007=CIRCLE('',#4744,0.5);
#1008=CIRCLE('',#4745,0.5);
#1009=CIRCLE('',#4747,7.95);
#1010=CIRCLE('',#4748,0.5);
#1011=CIRCLE('',#4750,0.5);
#1012=CIRCLE('',#4757,0.5);
#1013=CIRCLE('',#4758,0.5);
#1014=CIRCLE('',#4761,8.45);
#1015=CIRCLE('',#4762,0.5);
#1016=CIRCLE('',#4763,7.95);
#1017=CIRCLE('',#4765,19.9567770454363);
#1018=CIRCLE('',#4766,0.5);
#1019=CIRCLE('',#4767,20.0425817450355);
#1020=CIRCLE('',#4768,20.0425817450355);
#1021=CIRCLE('',#4771,51.);
#1022=CIRCLE('',#4772,51.);
#1023=CIRCLE('',#4774,0.5);
#1024=CIRCLE('',#4775,0.5);
#1025=CIRCLE('',#4778,0.5);
#1026=CIRCLE('',#4780,0.5);
#1027=CIRCLE('',#4784,0.499999999999991);
#1028=CIRCLE('',#4785,0.499999999999993);
#1029=CIRCLE('',#4787,0.5);
#1030=CIRCLE('',#4789,0.50000000000002);
#1031=CIRCLE('',#4791,0.5);
#1209=LINE('',#10478,#1439);
#1210=LINE('',#10481,#1440);
#1211=LINE('',#10484,#1441);
#1212=LINE('',#11012,#1442);
#1213=LINE('',#11138,#1443);
#1214=LINE('',#11150,#1444);
#1215=LINE('',#11154,#1445);
#1216=LINE('',#11155,#1446);
#1217=LINE('',#11159,#1447);
#1218=LINE('',#11164,#1448);
#1219=LINE('',#11168,#1449);
#1220=LINE('',#11180,#1450);
#1221=LINE('',#11183,#1451);
#1222=LINE('',#11186,#1452);
#1223=LINE('',#11187,#1453);
#1224=LINE('',#11190,#1454);
#1225=LINE('',#11191,#1455);
#1226=LINE('',#11196,#1456);
#1227=LINE('',#11203,#1457);
#1228=LINE('',#11219,#1458);
#1229=LINE('',#11222,#1459);
#1230=LINE('',#11231,#1460);
#1231=LINE('',#11235,#1461);
#1232=LINE('',#11236,#1462);
#1233=LINE('',#11240,#1463);
#1234=LINE('',#11375,#1464);
#1235=LINE('',#11720,#1465);
#1439=VECTOR('',#5512,10.);
#1440=VECTOR('',#5515,10.);
#1441=VECTOR('',#5518,10.);
#1442=VECTOR('',#5535,10.);
#1443=VECTOR('',#5542,35.);
#1444=VECTOR('',#5555,10.);
#1445=VECTOR('',#5558,10.);
#1446=VECTOR('',#5559,10.);
#1447=VECTOR('',#5564,12.);
#1448=VECTOR('',#5569,10.);
#1449=VECTOR('',#5574,10.);
#1450=VECTOR('',#5591,10.);
#1451=VECTOR('',#5594,10.);
#1452=VECTOR('',#5597,10.);
#1453=VECTOR('',#5598,10.);
#1454=VECTOR('',#5601,10.);
#1455=VECTOR('',#5602,10.);
#1456=VECTOR('',#5607,10.);
#1457=VECTOR('',#5618,10.);
#1458=VECTOR('',#5639,10.);
#1459=VECTOR('',#5642,35.5);
#1460=VECTOR('',#5655,10.);
#1461=VECTOR('',#5660,10.);
#1462=VECTOR('',#5661,10.);
#1463=VECTOR('',#5668,10.);
#1464=VECTOR('',#5679,10.);
#1465=VECTOR('',#5692,10.);
#1684=B_SPLINE_CURVE_WITH_KNOTS('',3,(#10431,#10432,#10433,#10434,#10435),
 .UNSPECIFIED.,.F.,.F.,(4,1,4),(0.,0.5,1.),.UNSPECIFIED.);
#1685=B_SPLINE_CURVE_WITH_KNOTS('',3,(#10439,#10440,#10441,#10442,#10443),
 .UNSPECIFIED.,.F.,.F.,(4,1,4),(0.,0.5,1.),.UNSPECIFIED.);
#1686=B_SPLINE_CURVE_WITH_KNOTS('',3,(#10466,#10467,#10468,#10469),
 .UNSPECIFIED.,.F.,.F.,(4,4),(0.088693979487329,0.125274232772668),
 .UNSPECIFIED.);
#1687=B_SPLINE_CURVE_WITH_KNOTS('',3,(#10472,#10473,#10474,#10475),
 .UNSPECIFIED.,.F.,.F.,(4,4),(-0.125274232772668,-0.088693979487329),
 .UNSPECIFIED.);
#1688=B_SPLINE_CURVE_WITH_KNOTS('',3,(#10485,#10486,#10487,#10488,#10489,
#10490,#10491,#10492,#10493,#10494,#10495,#10496,#10497,#10498,#10499,#10500,
#10501,#10502,#10503,#10504,#10505),.UNSPECIFIED.,.F.,.F.,(4,1,1,1,1,1,
1,1,1,1,1,1,1,1,1,1,1,1,4),(0.,2.5201892997592,5.0403785995184,6.72050479935786,
8.40063099919733,10.0807571990368,11.7608833988763,15.1211357985552,15.9611988984749,
16.8012619983947,20.1615143980736,21.841640597913,23.5217667977525,25.201892997592,
26.8820191974314,28.5621453972709,30.2422715971104,32.7624608968696,35.2826501966288),
 .UNSPECIFIED.);
#1689=B_SPLINE_CURVE_WITH_KNOTS('',3,(#10597,#10598,#10599,#10600,#10601,
#10602,#10603,#10604,#10605,#10606,#10607,#10608,#10609,#10610,#10611,#10612,
#10613,#10614,#10615,#10616,#10617,#10618),.UNSPECIFIED.,.F.,.F.,(4,1,1,
1,1,1,1,1,1,1,1,1,1,1,1,1,1,1,1,4),(-34.8725995211214,-32.381699555327,
-29.8907995895326,-28.2301996123364,-26.5695996351401,-24.9089996579439,
-23.2483996807476,-21.5877997035514,-19.9271997263551,-18.2665997491588,
-16.6059997719626,-14.9453997947663,-13.2847998175701,-11.6241998403738,
-9.96359986317755,-8.30299988598129,-6.64239990878503,-4.98179993158877,
-2.49089996579439,0.),.UNSPECIFIED.);
#1690=B_SPLINE_CURVE_WITH_KNOTS('',3,(#10621,#10622,#10623,#10624,#10625,
#10626,#10627,#10628,#10629,#10630,#10631,#10632,#10633,#10634,#10635,#10636,
#10637,#10638,#10639,#10640,#10641,#10642),.UNSPECIFIED.,.F.,.F.,(4,1,1,
1,1,1,1,1,1,1,1,1,1,1,1,1,1,1,1,4),(0.,2.49089996579439,4.98179993158877,
6.64239990878503,8.30299988598129,9.96359986317755,11.6241998403738,13.2847998175701,
14.9453997947663,16.6059997719626,18.2665997491588,19.9271997263551,21.5877997035514,
23.2483996807476,24.9089996579439,26.5695996351401,28.2301996123364,29.8907995895326,
32.381699555327,34.8725995211214),.UNSPECIFIED.);
#1691=B_SPLINE_CURVE_WITH_KNOTS('',3,(#10669,#10670,#10671,#10672),
 .UNSPECIFIED.,.F.,.F.,(4,4),(0.0886939794873267,0.125274232772633),
 .UNSPECIFIED.);
#1692=B_SPLINE_CURVE_WITH_KNOTS('',3,(#10673,#10674,#10675,#10676),
 .UNSPECIFIED.,.F.,.F.,(4,4),(-0.125274232772633,-0.0886939794873267),
 .UNSPECIFIED.);
#1693=B_SPLINE_CURVE_WITH_KNOTS('',3,(#10694,#10695,#10696,#10697),
 .UNSPECIFIED.,.F.,.F.,(4,4),(-0.860462555942468,-0.587131769179142),
 .UNSPECIFIED.);
#1694=B_SPLINE_CURVE_WITH_KNOTS('',3,(#10699,#10700,#10701,#10702,#10703,
#10704,#10705,#10706,#10707,#10708,#10709,#10710,#10711,#10712,#10713,#10714,
#10715,#10716,#10717,#10718,#10719,#10720,#10721,#10722,#10723),
 .UNSPECIFIED.,.F.,.F.,(4,3,3,3,3,3,3,3,4),(-0.000295685355657064,0.,0.010783911952954,
0.021297945774393,0.0312974952251527,0.034783930866502,0.0432659714995236,
0.0512040825193111,0.0584686894100284),.UNSPECIFIED.);
#1695=B_SPLINE_CURVE_WITH_KNOTS('',3,(#10725,#10726,#10727,#10728,#10729,
#10730),.UNSPECIFIED.,.F.,.F.,(4,2,4),(-0.0365164375971617,-0.026613618341596,
0.),.UNSPECIFIED.);
#1696=B_SPLINE_CURVE_WITH_KNOTS('',3,(#10731,#10732,#10733,#10734),
 .UNSPECIFIED.,.F.,.F.,(4,4),(0.649033397962949,0.860462555942468),
 .UNSPECIFIED.);
#1697=B_SPLINE_CURVE_WITH_KNOTS('',3,(#10916,#10917,#10918,#10919),
 .UNSPECIFIED.,.F.,.F.,(4,4),(-0.292336438831091,-0.0190073922957582),
 .UNSPECIFIED.);
#1698=B_SPLINE_CURVE_WITH_KNOTS('',3,(#10921,#10922,#10923,#10924),
 .UNSPECIFIED.,.F.,.F.,(4,4),(-34.9074997830359,-34.6574150541607),
 .UNSPECIFIED.);
#1699=B_SPLINE_CURVE_WITH_KNOTS('',3,(#10941,#10942,#10943,#10944,#10945,
#10946,#10947,#10948,#10949,#10950,#10951,#10952,#10953,#10954,#10955,#10956,
#10957,#10958,#10959,#10960,#10961,#10962,#10963),.UNSPECIFIED.,.T.,.F.,
(4,1,1,1,1,1,1,1,1,1,1,1,1,1,1,1,1,1,1,1,4),(-7.85398163397448,-7.40518268346166,
-6.95638373294883,-6.65718443260694,-6.35798513226506,-6.20838548209412,
-6.05878583192317,-5.75958653158129,-5.4603872312394,-5.16118793089752,
-4.86198863055563,-4.56278933021375,-4.26359002987186,-3.96439072952998,
-3.66519142918809,-3.36599212884621,-3.06679282850432,-2.76759352816244,
-2.46839422782055,-2.01959527730772,-1.5707963267949),.UNSPECIFIED.);
#1700=B_SPLINE_CURVE_WITH_KNOTS('',3,(#10964,#10965,#10966,#10967),
 .UNSPECIFIED.,.F.,.F.,(4,4),(-35.1575805274809,-34.9074997830359),
 .UNSPECIFIED.);
#1701=B_SPLINE_CURVE_WITH_KNOTS('',3,(#10985,#10986,#10987,#10988),
 .UNSPECIFIED.,.F.,.F.,(4,4),(0.0190073922957582,0.230436959265831),
 .UNSPECIFIED.);
#1702=B_SPLINE_CURVE_WITH_KNOTS('',3,(#10990,#10991,#10992,#10993,#10994,
#10995,#10996,#10997),.UNSPECIFIED.,.F.,.F.,(4,2,2,4),(-0.0846091546938526,
-0.070148598643786,-0.0557294988245446,-0.048303086999004),
 .UNSPECIFIED.);
#1703=B_SPLINE_CURVE_WITH_KNOTS('',3,(#10998,#10999,#11000,#11001,#11002,
#11003,#11004,#11005),.UNSPECIFIED.,.F.,.F.,(4,2,2,4),(-0.0583052907282766,
-0.0580119153510426,-0.0234997264609151,0.),.UNSPECIFIED.);
#1704=B_SPLINE_CURVE_WITH_KNOTS('',3,(#11008,#11009,#11010,#11011),
 .UNSPECIFIED.,.F.,.F.,(4,4),(0.875635390636623,1.1096475233552),
 .UNSPECIFIED.);
#1705=B_SPLINE_CURVE_WITH_KNOTS('',3,(#11108,#11109,#11110,#11111,#11112,
#11113,#11114,#11115,#11116,#11117,#11118,#11119,#11120),.UNSPECIFIED.,
 .F.,.F.,(4,1,1,1,1,1,1,1,1,1,4),(1.5707963267949,2.01959527730772,2.46839422782055,
2.76759352816244,3.06679282850432,3.36599212884621,3.66519142918809,3.96439072952998,
4.26359002987186,4.56278933021375,4.71238073889391),.UNSPECIFIED.);
#1706=B_SPLINE_CURVE_WITH_KNOTS('',3,(#11121,#11122,#11123,#11124,#11125,
#11126,#11127,#11128,#11129,#11130,#11131,#11132,#11133,#11134),
 .UNSPECIFIED.,.F.,.F.,(4,1,1,1,1,1,1,1,1,1,1,4),(4.71238073889391,4.86198863055563,
5.16118793089752,5.4603872312394,5.75958653158129,6.05878583192317,6.20838548209412,
6.35798513226506,6.65718443260694,6.95638373294883,7.40518268346166,7.85398163397448),
 .UNSPECIFIED.);
#1707=B_SPLINE_CURVE_WITH_KNOTS('',3,(#11351,#11352,#11353,#11354,#11355,
#11356,#11357,#11358,#11359,#11360,#11361,#11362,#11363,#11364,#11365,#11366,
#11367,#11368,#11369,#11370,#11371),.UNSPECIFIED.,.F.,.F.,(4,1,1,1,1,1,
1,1,1,1,1,1,1,1,1,1,1,1,4),(-35.2826501966288,-32.7624608968696,-30.2422715971104,
-28.5621453972709,-26.8820191974314,-25.201892997592,-23.5217667977525,
-21.841640597913,-20.1615143980736,-16.8012619983947,-15.9611988984749,
-15.1211357985552,-11.7608833988763,-10.0807571990368,-8.40063099919733,
-6.72050479935786,-5.0403785995184,-2.5201892997592,0.),.UNSPECIFIED.);
#1708=B_SPLINE_CURVE_WITH_KNOTS('',3,(#11398,#11399,#11400,#11401),
 .UNSPECIFIED.,.F.,.F.,(4,4),(-1.1096475233552,-0.825569897711632),
 .UNSPECIFIED.);
#1709=B_SPLINE_CURVE_WITH_KNOTS('',3,(#11403,#11404,#11405,#11406,#11407,
#11408,#11409,#11410,#11411,#11412,#11413,#11414,#11415,#11416),
 .UNSPECIFIED.,.F.,.F.,(4,2,2,2,2,2,4),(-0.0987748436415996,-0.0846442489344777,
-0.0686516240192571,-0.0476703451541984,-0.0244527973261725,0.,0.00045791775862737),
 .UNSPECIFIED.);
#1710=B_SPLINE_CURVE_WITH_KNOTS('',3,(#11417,#11418,#11419,#11420),
 .UNSPECIFIED.,.F.,.F.,(4,4),(-0.000473389988960978,0.),.UNSPECIFIED.);
#1711=B_SPLINE_CURVE_WITH_KNOTS('',3,(#11647,#11648,#11649,#11650),
 .UNSPECIFIED.,.F.,.F.,(4,4),(-0.317361133028268,-0.0332835073847237),
 .UNSPECIFIED.);
#1712=B_SPLINE_CURVE_WITH_KNOTS('',3,(#11652,#11653,#11654,#11655),
 .UNSPECIFIED.,.F.,.F.,(4,4),(-36.1074649321654,-35.8573857487427),
 .UNSPECIFIED.);
#1713=B_SPLINE_CURVE_WITH_KNOTS('',3,(#11675,#11676,#11677,#11678),
 .UNSPECIFIED.,.F.,.F.,(4,4),(-36.3575403182,-36.1074649321654),
 .UNSPECIFIED.);
#1714=B_SPLINE_CURVE_WITH_KNOTS('',3,(#11696,#11697,#11698,#11699),
 .UNSPECIFIED.,.F.,.F.,(4,4),(0.0332835073847237,0.267295640103291),
 .UNSPECIFIED.);
#1715=B_SPLINE_CURVE_WITH_KNOTS('',3,(#11701,#11702,#11703,#11704),
 .UNSPECIFIED.,.F.,.F.,(4,4),(-0.0809288342320163,-0.0804554916472578),
 .UNSPECIFIED.);
#1716=B_SPLINE_CURVE_WITH_KNOTS('',3,(#11705,#11706,#11707,#11708,#11709,
#11710,#11711,#11712,#11713,#11714,#11715,#11716,#11717,#11718),
 .UNSPECIFIED.,.F.,.F.,(4,2,2,2,2,2,4),(0.,0.0139873855694353,0.0298179302556126,
0.0505865704508789,0.0735688157275276,0.0977737916359578,0.0982270685416762),
 .UNSPECIFIED.);
#1717=B_SPLINE_CURVE_WITH_KNOTS('',3,(#11738,#11739,#11740,#11741),
 .UNSPECIFIED.,.F.,.F.,(4,4),(34.6979587163218,34.7074565752905),
 .UNSPECIFIED.);
#1718=B_SPLINE_CURVE_WITH_KNOTS('',3,(#11743,#11744,#11745,#11746),
 .UNSPECIFIED.,.F.,.F.,(4,4),(34.7074565752905,35.1075404676718),
 .UNSPECIFIED.);
#1719=B_SPLINE_CURVE_WITH_KNOTS('',3,(#11747,#11748,#11749,#11750),
 .UNSPECIFIED.,.F.,.F.,(4,4),(-35.1170380704337,-35.1075404676718),
 .UNSPECIFIED.);
#1720=B_SPLINE_CURVE_WITH_KNOTS('',3,(#11753,#11754,#11755,#11756),
 .UNSPECIFIED.,.F.,.F.,(4,4),(36.3075029101841,36.3075051513331),
 .UNSPECIFIED.);
#1721=B_SPLINE_CURVE_WITH_KNOTS('',3,(#11758,#11759,#11760,#11761),
 .UNSPECIFIED.,.F.,.F.,(4,4),(35.9074245478542,36.3075029101841),
 .UNSPECIFIED.);
#1722=B_SPLINE_CURVE_WITH_KNOTS('',3,(#11762,#11763,#11764,#11765),
 .UNSPECIFIED.,.F.,.F.,(4,4),(-35.9074245478542,-35.9074223066489),
 .UNSPECIFIED.);
#1927=VERTEX_POINT('',#10421);
#1928=VERTEX_POINT('',#10422);
#1929=VERTEX_POINT('',#10424);
#1930=VERTEX_POINT('',#10426);
#1931=VERTEX_POINT('',#10430);
#1932=VERTEX_POINT('',#10438);
#1933=VERTEX_POINT('',#10465);
#1934=VERTEX_POINT('',#10470);
#1935=VERTEX_POINT('',#10477);
#1936=VERTEX_POINT('',#10479);
#1937=VERTEX_POINT('',#10483);
#1938=VERTEX_POINT('',#10594);
#1939=VERTEX_POINT('',#10595);
#1940=VERTEX_POINT('',#10619);
#1941=VERTEX_POINT('',#10644);
#1942=VERTEX_POINT('',#10693);
#1943=VERTEX_POINT('',#10698);
#1944=VERTEX_POINT('',#10724);
#1945=VERTEX_POINT('',#10915);
#1946=VERTEX_POINT('',#10920);
#1947=VERTEX_POINT('',#10925);
#1948=VERTEX_POINT('',#10984);
#1949=VERTEX_POINT('',#10989);
#1950=VERTEX_POINT('',#11007);
#1951=VERTEX_POINT('',#11105);
#1952=VERTEX_POINT('',#11107);
#1953=VERTEX_POINT('',#11136);
#1954=VERTEX_POINT('',#11140);
#1955=VERTEX_POINT('',#11141);
#1956=VERTEX_POINT('',#11144);
#1957=VERTEX_POINT('',#11148);
#1958=VERTEX_POINT('',#11149);
#1959=VERTEX_POINT('',#11151);
#1960=VERTEX_POINT('',#11153);
#1961=VERTEX_POINT('',#11157);
#1962=VERTEX_POINT('',#11161);
#1963=VERTEX_POINT('',#11163);
#1964=VERTEX_POINT('',#11167);
#1965=VERTEX_POINT('',#11171);
#1966=VERTEX_POINT('',#11175);
#1967=VERTEX_POINT('',#11179);
#1968=VERTEX_POINT('',#11181);
#1969=VERTEX_POINT('',#11185);
#1970=VERTEX_POINT('',#11189);
#1971=VERTEX_POINT('',#11193);
#1972=VERTEX_POINT('',#11195);
#1973=VERTEX_POINT('',#11199);
#1974=VERTEX_POINT('',#11205);
#1975=VERTEX_POINT('',#11207);
#1976=VERTEX_POINT('',#11211);
#1977=VERTEX_POINT('',#11213);
#1978=VERTEX_POINT('',#11215);
#1979=VERTEX_POINT('',#11221);
#1980=VERTEX_POINT('',#11223);
#1981=VERTEX_POINT('',#11227);
#1982=VERTEX_POINT('',#11233);
#1983=VERTEX_POINT('',#11348);
#1984=VERTEX_POINT('',#11350);
#1985=VERTEX_POINT('',#11374);
#1986=VERTEX_POINT('',#11397);
#1987=VERTEX_POINT('',#11402);
#1988=VERTEX_POINT('',#11646);
#1989=VERTEX_POINT('',#11651);
#1990=VERTEX_POINT('',#11695);
#1991=VERTEX_POINT('',#11700);
#1992=VERTEX_POINT('',#11737);
#1993=VERTEX_POINT('',#11742);
#1994=VERTEX_POINT('',#11752);
#1995=VERTEX_POINT('',#11757);
#2418=EDGE_CURVE('',#1927,#1928,#985,.T.);
#2419=EDGE_CURVE('',#1928,#1929,#986,.T.);
#2420=EDGE_CURVE('',#1929,#1930,#987,.T.);
#2421=EDGE_CURVE('',#1930,#1927,#988,.T.);
#2422=EDGE_CURVE('',#1929,#1931,#1684,.T.);
#2423=EDGE_CURVE('',#1931,#1930,#989,.T.);
#2424=EDGE_CURVE('',#1932,#1928,#1685,.T.);
#2425=EDGE_CURVE('',#1927,#1932,#990,.T.);
#2426=EDGE_CURVE('',#1932,#1933,#1686,.T.);
#2427=EDGE_CURVE('',#1934,#1933,#991,.T.);
#2428=EDGE_CURVE('',#1934,#1928,#1687,.T.);
#2429=EDGE_CURVE('',#1927,#1935,#1209,.T.);
#2430=EDGE_CURVE('',#1935,#1936,#992,.T.);
#2431=EDGE_CURVE('',#1936,#1932,#1210,.T.);
#2432=EDGE_CURVE('',#1937,#1930,#1211,.T.);
#2433=EDGE_CURVE('',#1935,#1937,#1688,.T.);
#2434=EDGE_CURVE('',#1938,#1939,#993,.T.);
#2435=EDGE_CURVE('',#1939,#1934,#1689,.T.);
#2436=EDGE_CURVE('',#1934,#1940,#994,.T.);
#2437=EDGE_CURVE('',#1940,#1938,#1690,.T.);
#2438=EDGE_CURVE('',#1938,#1941,#995,.T.);
#2439=EDGE_CURVE('',#1941,#1939,#996,.T.);
#2440=EDGE_CURVE('',#1933,#1940,#997,.T.);
#2441=EDGE_CURVE('',#1929,#1939,#1691,.T.);
#2442=EDGE_CURVE('',#1941,#1931,#1692,.T.);
#2443=EDGE_CURVE('',#1938,#1942,#1693,.T.);
#2444=EDGE_CURVE('',#1942,#1943,#1694,.T.);
#2445=EDGE_CURVE('',#1943,#1944,#1695,.T.);
#2446=EDGE_CURVE('',#1944,#1941,#1696,.T.);
#2447=EDGE_CURVE('',#1945,#1940,#1697,.T.);
#2448=EDGE_CURVE('',#1946,#1945,#1698,.T.);
#2449=EDGE_CURVE('',#1947,#1946,#292,.T.);
#2450=EDGE_CURVE('',#1947,#1947,#1699,.T.);
#2451=EDGE_CURVE('',#1942,#1946,#1700,.T.);
#2452=EDGE_CURVE('',#1933,#1948,#1701,.T.);
#2453=EDGE_CURVE('',#1948,#1949,#1702,.T.);
#2454=EDGE_CURVE('',#1945,#1949,#1703,.T.);
#2455=EDGE_CURVE('',#1950,#1936,#1704,.T.);
#2456=EDGE_CURVE('',#1948,#1950,#1212,.T.);
#2457=EDGE_CURVE('',#1947,#1951,#998,.T.);
#2458=EDGE_CURVE('',#1951,#1952,#1705,.T.);
#2459=EDGE_CURVE('',#1952,#1951,#1706,.T.);
#2460=EDGE_CURVE('',#1953,#1953,#999,.T.);
#2461=EDGE_CURVE('',#1953,#1952,#1213,.T.);
#2462=EDGE_CURVE('',#1954,#1955,#1000,.T.);
#2463=EDGE_CURVE('',#1955,#1954,#1001,.T.);
#2464=EDGE_CURVE('',#1954,#1956,#1002,.T.);
#2465=EDGE_CURVE('',#1956,#1956,#1003,.T.);
#2466=EDGE_CURVE('',#1957,#1958,#1214,.T.);
#2467=EDGE_CURVE('',#1959,#1957,#1004,.T.);
#2468=EDGE_CURVE('',#1960,#1959,#1215,.T.);
#2469=EDGE_CURVE('',#1958,#1960,#1216,.T.);
#2470=EDGE_CURVE('',#1961,#1961,#1005,.T.);
#2471=EDGE_CURVE('',#1961,#1955,#1217,.T.);
#2472=EDGE_CURVE('',#1960,#1962,#63,.F.);
#2473=EDGE_CURVE('',#1962,#1963,#1218,.T.);
#2474=EDGE_CURVE('',#1963,#1958,#64,.T.);
#2475=EDGE_CURVE('',#1963,#1964,#1219,.T.);
#2476=EDGE_CURVE('',#1964,#1957,#1006,.T.);
#2477=EDGE_CURVE('',#1964,#1965,#1007,.T.);
#2478=EDGE_CURVE('',#1965,#1957,#1008,.T.);
#2479=EDGE_CURVE('',#1965,#1966,#1009,.T.);
#2480=EDGE_CURVE('',#1966,#1959,#1010,.F.);
#2481=EDGE_CURVE('',#1964,#1967,#1220,.T.);
#2482=EDGE_CURVE('',#1968,#1967,#1011,.T.);
#2483=EDGE_CURVE('',#1968,#1965,#1221,.T.);
#2484=EDGE_CURVE('',#1969,#1963,#1222,.T.);
#2485=EDGE_CURVE('',#1967,#1969,#1223,.T.);
#2486=EDGE_CURVE('',#1962,#1970,#1224,.T.);
#2487=EDGE_CURVE('',#1969,#1970,#1225,.T.);
#2488=EDGE_CURVE('',#1970,#1971,#65,.F.);
#2489=EDGE_CURVE('',#1971,#1972,#1226,.T.);
#2490=EDGE_CURVE('',#1972,#1969,#66,.T.);
#2491=EDGE_CURVE('',#1967,#1973,#1012,.T.);
#2492=EDGE_CURVE('',#1973,#1968,#1013,.T.);
#2493=EDGE_CURVE('',#1972,#1973,#1227,.T.);
#2494=EDGE_CURVE('',#1973,#1974,#1014,.T.);
#2495=EDGE_CURVE('',#1974,#1975,#1015,.T.);
#2496=EDGE_CURVE('',#1975,#1968,#1016,.T.);
#2497=EDGE_CURVE('',#1976,#1976,#1017,.T.);
#2498=EDGE_CURVE('',#1976,#1977,#1018,.T.);
#2499=EDGE_CURVE('',#1977,#1978,#1019,.T.);
#2500=EDGE_CURVE('',#1978,#1977,#1020,.T.);
#2501=EDGE_CURVE('',#1974,#1971,#1228,.T.);
#2502=EDGE_CURVE('',#1978,#1979,#1229,.T.);
#2503=EDGE_CURVE('',#1979,#1980,#1021,.T.);
#2504=EDGE_CURVE('',#1980,#1979,#1022,.T.);
#2505=EDGE_CURVE('',#1981,#1966,#1023,.F.);
#2506=EDGE_CURVE('',#1959,#1981,#1024,.F.);
#2507=EDGE_CURVE('',#1981,#1962,#1230,.T.);
#2508=EDGE_CURVE('',#1975,#1982,#1025,.T.);
#2509=EDGE_CURVE('',#1982,#1981,#1231,.T.);
#2510=EDGE_CURVE('',#1966,#1975,#1232,.T.);
#2511=EDGE_CURVE('',#1974,#1982,#1026,.T.);
#2512=EDGE_CURVE('',#1970,#1982,#1233,.T.);
#2513=EDGE_CURVE('',#1937,#1983,#1027,.T.);
#2514=EDGE_CURVE('',#1983,#1984,#1707,.T.);
#2515=EDGE_CURVE('',#1984,#1935,#1028,.T.);
#2516=EDGE_CURVE('',#1931,#1985,#1234,.T.);
#2517=EDGE_CURVE('',#1985,#1937,#1029,.T.);
#2518=EDGE_CURVE('',#1985,#1983,#1030,.T.);
#2519=EDGE_CURVE('',#1984,#1936,#1031,.T.);
#2520=EDGE_CURVE('',#1984,#1986,#1708,.T.);
#2521=EDGE_CURVE('',#1987,#1986,#1709,.T.);
#2522=EDGE_CURVE('',#1987,#1950,#1710,.T.);
#2523=EDGE_CURVE('',#1988,#1983,#1711,.T.);
#2524=EDGE_CURVE('',#1989,#1988,#1712,.T.);
#2525=EDGE_CURVE('',#1989,#1980,#293,.T.);
#2526=EDGE_CURVE('',#1986,#1989,#1713,.T.);
#2527=EDGE_CURVE('',#1985,#1990,#1714,.T.);
#2528=EDGE_CURVE('',#1990,#1991,#1715,.T.);
#2529=EDGE_CURVE('',#1991,#1988,#1716,.T.);
#2530=EDGE_CURVE('',#1990,#1944,#1235,.T.);
#2531=EDGE_CURVE('',#1949,#1992,#1717,.T.);
#2532=EDGE_CURVE('',#1992,#1993,#1718,.T.);
#2533=EDGE_CURVE('',#1943,#1993,#1719,.T.);
#2534=EDGE_CURVE('',#1994,#1987,#1720,.T.);
#2535=EDGE_CURVE('',#1995,#1994,#1721,.T.);
#2536=EDGE_CURVE('',#1995,#1991,#1722,.T.);
#3331=ORIENTED_EDGE('',*,*,#2418,.T.);
#3332=ORIENTED_EDGE('',*,*,#2419,.T.);
#3333=ORIENTED_EDGE('',*,*,#2420,.T.);
#3334=ORIENTED_EDGE('',*,*,#2421,.T.);
#3335=ORIENTED_EDGE('',*,*,#2422,.T.);
#3336=ORIENTED_EDGE('',*,*,#2423,.T.);
#3337=ORIENTED_EDGE('',*,*,#2420,.F.);
#3338=ORIENTED_EDGE('',*,*,#2424,.T.);
#3339=ORIENTED_EDGE('',*,*,#2418,.F.);
#3340=ORIENTED_EDGE('',*,*,#2425,.T.);
#3341=ORIENTED_EDGE('',*,*,#2424,.F.);
#3342=ORIENTED_EDGE('',*,*,#2426,.T.);
#3343=ORIENTED_EDGE('',*,*,#2427,.F.);
#3344=ORIENTED_EDGE('',*,*,#2428,.T.);
#3345=ORIENTED_EDGE('',*,*,#2425,.F.);
#3346=ORIENTED_EDGE('',*,*,#2429,.T.);
#3347=ORIENTED_EDGE('',*,*,#2430,.T.);
#3348=ORIENTED_EDGE('',*,*,#2431,.T.);
#3349=ORIENTED_EDGE('',*,*,#2421,.F.);
#3350=ORIENTED_EDGE('',*,*,#2432,.F.);
#3351=ORIENTED_EDGE('',*,*,#2433,.F.);
#3352=ORIENTED_EDGE('',*,*,#2429,.F.);
#3353=ORIENTED_EDGE('',*,*,#2434,.T.);
#3354=ORIENTED_EDGE('',*,*,#2435,.T.);
#3355=ORIENTED_EDGE('',*,*,#2436,.T.);
#3356=ORIENTED_EDGE('',*,*,#2437,.T.);
#3357=ORIENTED_EDGE('',*,*,#2434,.F.);
#3358=ORIENTED_EDGE('',*,*,#2438,.T.);
#3359=ORIENTED_EDGE('',*,*,#2439,.T.);
#3360=ORIENTED_EDGE('',*,*,#2427,.T.);
#3361=ORIENTED_EDGE('',*,*,#2440,.T.);
#3362=ORIENTED_EDGE('',*,*,#2436,.F.);
#3363=ORIENTED_EDGE('',*,*,#2422,.F.);
#3364=ORIENTED_EDGE('',*,*,#2441,.T.);
#3365=ORIENTED_EDGE('',*,*,#2439,.F.);
#3366=ORIENTED_EDGE('',*,*,#2442,.T.);
#3367=ORIENTED_EDGE('',*,*,#2438,.F.);
#3368=ORIENTED_EDGE('',*,*,#2443,.T.);
#3369=ORIENTED_EDGE('',*,*,#2444,.T.);
#3370=ORIENTED_EDGE('',*,*,#2445,.T.);
#3371=ORIENTED_EDGE('',*,*,#2446,.T.);
#3372=ORIENTED_EDGE('',*,*,#2437,.F.);
#3373=ORIENTED_EDGE('',*,*,#2447,.F.);
#3374=ORIENTED_EDGE('',*,*,#2448,.F.);
#3375=ORIENTED_EDGE('',*,*,#2449,.F.);
#3376=ORIENTED_EDGE('',*,*,#2450,.F.);
#3377=ORIENTED_EDGE('',*,*,#2449,.T.);
#3378=ORIENTED_EDGE('',*,*,#2451,.F.);
#3379=ORIENTED_EDGE('',*,*,#2443,.F.);
#3380=ORIENTED_EDGE('',*,*,#2440,.F.);
#3381=ORIENTED_EDGE('',*,*,#2452,.T.);
#3382=ORIENTED_EDGE('',*,*,#2453,.T.);
#3383=ORIENTED_EDGE('',*,*,#2454,.F.);
#3384=ORIENTED_EDGE('',*,*,#2447,.T.);
#3385=ORIENTED_EDGE('',*,*,#2426,.F.);
#3386=ORIENTED_EDGE('',*,*,#2431,.F.);
#3387=ORIENTED_EDGE('',*,*,#2455,.F.);
#3388=ORIENTED_EDGE('',*,*,#2456,.F.);
#3389=ORIENTED_EDGE('',*,*,#2452,.F.);
#3390=ORIENTED_EDGE('',*,*,#2457,.T.);
#3391=ORIENTED_EDGE('',*,*,#2458,.T.);
#3392=ORIENTED_EDGE('',*,*,#2459,.T.);
#3393=ORIENTED_EDGE('',*,*,#2457,.F.);
#3394=ORIENTED_EDGE('',*,*,#2450,.T.);
#3395=ORIENTED_EDGE('',*,*,#2460,.T.);
#3396=ORIENTED_EDGE('',*,*,#2461,.T.);
#3397=ORIENTED_EDGE('',*,*,#2458,.F.);
#3398=ORIENTED_EDGE('',*,*,#2459,.F.);
#3399=ORIENTED_EDGE('',*,*,#2461,.F.);
#3400=ORIENTED_EDGE('',*,*,#2462,.T.);
#3401=ORIENTED_EDGE('',*,*,#2463,.T.);
#3402=ORIENTED_EDGE('',*,*,#2464,.T.);
#3403=ORIENTED_EDGE('',*,*,#2465,.T.);
#3404=ORIENTED_EDGE('',*,*,#2464,.F.);
#3405=ORIENTED_EDGE('',*,*,#2465,.F.);
#3406=ORIENTED_EDGE('',*,*,#2466,.F.);
#3407=ORIENTED_EDGE('',*,*,#2467,.F.);
#3408=ORIENTED_EDGE('',*,*,#2468,.F.);
#3409=ORIENTED_EDGE('',*,*,#2469,.F.);
#3410=ORIENTED_EDGE('',*,*,#2470,.F.);
#3411=ORIENTED_EDGE('',*,*,#2471,.T.);
#3412=ORIENTED_EDGE('',*,*,#2462,.F.);
#3413=ORIENTED_EDGE('',*,*,#2463,.F.);
#3414=ORIENTED_EDGE('',*,*,#2471,.F.);
#3415=ORIENTED_EDGE('',*,*,#2469,.T.);
#3416=ORIENTED_EDGE('',*,*,#2472,.T.);
#3417=ORIENTED_EDGE('',*,*,#2473,.T.);
#3418=ORIENTED_EDGE('',*,*,#2474,.T.);
#3419=ORIENTED_EDGE('',*,*,#2475,.T.);
#3420=ORIENTED_EDGE('',*,*,#2476,.T.);
#3421=ORIENTED_EDGE('',*,*,#2466,.T.);
#3422=ORIENTED_EDGE('',*,*,#2474,.F.);
#3423=ORIENTED_EDGE('',*,*,#2476,.F.);
#3424=ORIENTED_EDGE('',*,*,#2477,.T.);
#3425=ORIENTED_EDGE('',*,*,#2478,.T.);
#3426=ORIENTED_EDGE('',*,*,#2478,.F.);
#3427=ORIENTED_EDGE('',*,*,#2479,.T.);
#3428=ORIENTED_EDGE('',*,*,#2480,.T.);
#3429=ORIENTED_EDGE('',*,*,#2467,.T.);
#3430=ORIENTED_EDGE('',*,*,#2477,.F.);
#3431=ORIENTED_EDGE('',*,*,#2481,.T.);
#3432=ORIENTED_EDGE('',*,*,#2482,.F.);
#3433=ORIENTED_EDGE('',*,*,#2483,.T.);
#3434=ORIENTED_EDGE('',*,*,#2475,.F.);
#3435=ORIENTED_EDGE('',*,*,#2484,.F.);
#3436=ORIENTED_EDGE('',*,*,#2485,.F.);
#3437=ORIENTED_EDGE('',*,*,#2481,.F.);
#3438=ORIENTED_EDGE('',*,*,#2473,.F.);
#3439=ORIENTED_EDGE('',*,*,#2486,.T.);
#3440=ORIENTED_EDGE('',*,*,#2487,.F.);
#3441=ORIENTED_EDGE('',*,*,#2484,.T.);
#3442=ORIENTED_EDGE('',*,*,#2487,.T.);
#3443=ORIENTED_EDGE('',*,*,#2488,.T.);
#3444=ORIENTED_EDGE('',*,*,#2489,.T.);
#3445=ORIENTED_EDGE('',*,*,#2490,.T.);
#3446=ORIENTED_EDGE('',*,*,#2491,.T.);
#3447=ORIENTED_EDGE('',*,*,#2492,.T.);
#3448=ORIENTED_EDGE('',*,*,#2482,.T.);
#3449=ORIENTED_EDGE('',*,*,#2493,.T.);
#3450=ORIENTED_EDGE('',*,*,#2491,.F.);
#3451=ORIENTED_EDGE('',*,*,#2485,.T.);
#3452=ORIENTED_EDGE('',*,*,#2490,.F.);
#3453=ORIENTED_EDGE('',*,*,#2492,.F.);
#3454=ORIENTED_EDGE('',*,*,#2494,.T.);
#3455=ORIENTED_EDGE('',*,*,#2495,.T.);
#3456=ORIENTED_EDGE('',*,*,#2496,.T.);
#3457=ORIENTED_EDGE('',*,*,#2497,.T.);
#3458=ORIENTED_EDGE('',*,*,#2498,.T.);
#3459=ORIENTED_EDGE('',*,*,#2499,.T.);
#3460=ORIENTED_EDGE('',*,*,#2500,.T.);
#3461=ORIENTED_EDGE('',*,*,#2498,.F.);
#3462=ORIENTED_EDGE('',*,*,#2497,.F.);
#3463=ORIENTED_EDGE('',*,*,#2501,.F.);
#3464=ORIENTED_EDGE('',*,*,#2494,.F.);
#3465=ORIENTED_EDGE('',*,*,#2493,.F.);
#3466=ORIENTED_EDGE('',*,*,#2489,.F.);
#3467=ORIENTED_EDGE('',*,*,#2500,.F.);
#3468=ORIENTED_EDGE('',*,*,#2502,.T.);
#3469=ORIENTED_EDGE('',*,*,#2503,.T.);
#3470=ORIENTED_EDGE('',*,*,#2504,.T.);
#3471=ORIENTED_EDGE('',*,*,#2502,.F.);
#3472=ORIENTED_EDGE('',*,*,#2499,.F.);
#3473=ORIENTED_EDGE('',*,*,#2505,.F.);
#3474=ORIENTED_EDGE('',*,*,#2506,.F.);
#3475=ORIENTED_EDGE('',*,*,#2480,.F.);
#3476=ORIENTED_EDGE('',*,*,#2468,.T.);
#3477=ORIENTED_EDGE('',*,*,#2506,.T.);
#3478=ORIENTED_EDGE('',*,*,#2507,.T.);
#3479=ORIENTED_EDGE('',*,*,#2472,.F.);
#3480=ORIENTED_EDGE('',*,*,#2508,.T.);
#3481=ORIENTED_EDGE('',*,*,#2509,.T.);
#3482=ORIENTED_EDGE('',*,*,#2505,.T.);
#3483=ORIENTED_EDGE('',*,*,#2510,.T.);
#3484=ORIENTED_EDGE('',*,*,#2495,.F.);
#3485=ORIENTED_EDGE('',*,*,#2511,.T.);
#3486=ORIENTED_EDGE('',*,*,#2508,.F.);
#3487=ORIENTED_EDGE('',*,*,#2507,.F.);
#3488=ORIENTED_EDGE('',*,*,#2509,.F.);
#3489=ORIENTED_EDGE('',*,*,#2512,.F.);
#3490=ORIENTED_EDGE('',*,*,#2486,.F.);
#3491=ORIENTED_EDGE('',*,*,#2511,.F.);
#3492=ORIENTED_EDGE('',*,*,#2501,.T.);
#3493=ORIENTED_EDGE('',*,*,#2488,.F.);
#3494=ORIENTED_EDGE('',*,*,#2512,.T.);
#3495=ORIENTED_EDGE('',*,*,#2496,.F.);
#3496=ORIENTED_EDGE('',*,*,#2510,.F.);
#3497=ORIENTED_EDGE('',*,*,#2479,.F.);
#3498=ORIENTED_EDGE('',*,*,#2483,.F.);
#3499=ORIENTED_EDGE('',*,*,#2513,.T.);
#3500=ORIENTED_EDGE('',*,*,#2514,.T.);
#3501=ORIENTED_EDGE('',*,*,#2515,.T.);
#3502=ORIENTED_EDGE('',*,*,#2433,.T.);
#3503=ORIENTED_EDGE('',*,*,#2423,.F.);
#3504=ORIENTED_EDGE('',*,*,#2516,.T.);
#3505=ORIENTED_EDGE('',*,*,#2517,.T.);
#3506=ORIENTED_EDGE('',*,*,#2432,.T.);
#3507=ORIENTED_EDGE('',*,*,#2517,.F.);
#3508=ORIENTED_EDGE('',*,*,#2518,.T.);
#3509=ORIENTED_EDGE('',*,*,#2513,.F.);
#3510=ORIENTED_EDGE('',*,*,#2515,.F.);
#3511=ORIENTED_EDGE('',*,*,#2519,.T.);
#3512=ORIENTED_EDGE('',*,*,#2430,.F.);
#3513=ORIENTED_EDGE('',*,*,#2519,.F.);
#3514=ORIENTED_EDGE('',*,*,#2520,.T.);
#3515=ORIENTED_EDGE('',*,*,#2521,.F.);
#3516=ORIENTED_EDGE('',*,*,#2522,.T.);
#3517=ORIENTED_EDGE('',*,*,#2455,.T.);
#3518=ORIENTED_EDGE('',*,*,#2514,.F.);
#3519=ORIENTED_EDGE('',*,*,#2523,.F.);
#3520=ORIENTED_EDGE('',*,*,#2524,.F.);
#3521=ORIENTED_EDGE('',*,*,#2525,.T.);
#3522=ORIENTED_EDGE('',*,*,#2503,.F.);
#3523=ORIENTED_EDGE('',*,*,#2504,.F.);
#3524=ORIENTED_EDGE('',*,*,#2525,.F.);
#3525=ORIENTED_EDGE('',*,*,#2526,.F.);
#3526=ORIENTED_EDGE('',*,*,#2520,.F.);
#3527=ORIENTED_EDGE('',*,*,#2518,.F.);
#3528=ORIENTED_EDGE('',*,*,#2527,.T.);
#3529=ORIENTED_EDGE('',*,*,#2528,.T.);
#3530=ORIENTED_EDGE('',*,*,#2529,.T.);
#3531=ORIENTED_EDGE('',*,*,#2523,.T.);
#3532=ORIENTED_EDGE('',*,*,#2442,.F.);
#3533=ORIENTED_EDGE('',*,*,#2446,.F.);
#3534=ORIENTED_EDGE('',*,*,#2530,.F.);
#3535=ORIENTED_EDGE('',*,*,#2527,.F.);
#3536=ORIENTED_EDGE('',*,*,#2516,.F.);
#3537=ORIENTED_EDGE('',*,*,#2451,.T.);
#3538=ORIENTED_EDGE('',*,*,#2448,.T.);
#3539=ORIENTED_EDGE('',*,*,#2454,.T.);
#3540=ORIENTED_EDGE('',*,*,#2531,.T.);
#3541=ORIENTED_EDGE('',*,*,#2532,.T.);
#3542=ORIENTED_EDGE('',*,*,#2533,.F.);
#3543=ORIENTED_EDGE('',*,*,#2444,.F.);
#3544=ORIENTED_EDGE('',*,*,#2532,.F.);
#3545=ORIENTED_EDGE('',*,*,#2531,.F.);
#3546=ORIENTED_EDGE('',*,*,#2453,.F.);
#3547=ORIENTED_EDGE('',*,*,#2456,.T.);
#3548=ORIENTED_EDGE('',*,*,#2522,.F.);
#3549=ORIENTED_EDGE('',*,*,#2534,.F.);
#3550=ORIENTED_EDGE('',*,*,#2535,.F.);
#3551=ORIENTED_EDGE('',*,*,#2536,.T.);
#3552=ORIENTED_EDGE('',*,*,#2528,.F.);
#3553=ORIENTED_EDGE('',*,*,#2530,.T.);
#3554=ORIENTED_EDGE('',*,*,#2445,.F.);
#3555=ORIENTED_EDGE('',*,*,#2533,.T.);
#3556=ORIENTED_EDGE('',*,*,#2535,.T.);
#3557=ORIENTED_EDGE('',*,*,#2534,.T.);
#3558=ORIENTED_EDGE('',*,*,#2521,.T.);
#3559=ORIENTED_EDGE('',*,*,#2526,.T.);
#3560=ORIENTED_EDGE('',*,*,#2524,.T.);
#3561=ORIENTED_EDGE('',*,*,#2529,.F.);
#3562=ORIENTED_EDGE('',*,*,#2536,.F.);
#3563=ORIENTED_EDGE('',*,*,#2460,.F.);
#3564=ORIENTED_EDGE('',*,*,#2470,.T.);
#3565=ORIENTED_EDGE('',*,*,#2419,.F.);
#3566=ORIENTED_EDGE('',*,*,#2428,.F.);
#3567=ORIENTED_EDGE('',*,*,#2435,.F.);
#3568=ORIENTED_EDGE('',*,*,#2441,.F.);
#4082=CYLINDRICAL_SURFACE('',#4715,0.5);
#4083=CYLINDRICAL_SURFACE('',#4736,12.);
#4084=CYLINDRICAL_SURFACE('',#4738,0.5);
#4085=CYLINDRICAL_SURFACE('',#4741,0.5);
#4086=CYLINDRICAL_SURFACE('',#4749,0.5);
#4087=CYLINDRICAL_SURFACE('',#4753,0.5);
#4088=CYLINDRICAL_SURFACE('',#4759,0.5);
#4089=CYLINDRICAL_SURFACE('',#4776,0.5);
#4090=CYLINDRICAL_SURFACE('',#4777,0.5);
#4091=CYLINDRICAL_SURFACE('',#4782,0.5);
#4092=CYLINDRICAL_SURFACE('',#4783,7.95);
#4093=CYLINDRICAL_SURFACE('',#4786,0.5);
#4228=ADVANCED_FACE('',(#438),#272,.T.);
#4229=ADVANCED_FACE('',(#439),#67,.T.);
#4230=ADVANCED_FACE('',(#440),#68,.T.);
#4231=ADVANCED_FACE('',(#441),#308,.F.);
#4232=ADVANCED_FACE('',(#442),#4082,.T.);
#4233=ADVANCED_FACE('',(#443),#196,.T.);
#4234=ADVANCED_FACE('',(#444),#309,.F.);
#4235=ADVANCED_FACE('',(#445),#69,.T.);
#4236=ADVANCED_FACE('',(#446),#70,.T.);
#4237=ADVANCED_FACE('',(#447),#310,.F.);
#4238=ADVANCED_FACE('',(#448),#311,.F.);
#4239=ADVANCED_FACE('',(#449),#296,.T.);
#4240=ADVANCED_FACE('',(#450),#312,.F.);
#4241=ADVANCED_FACE('',(#451),#197,.F.);
#4242=ADVANCED_FACE('',(#452),#313,.F.);
#4243=ADVANCED_FACE('',(#453),#89,.F.);
#4244=ADVANCED_FACE('',(#454),#273,.T.);
#4245=ADVANCED_FACE('',(#455,#153),#198,.T.);
#4246=ADVANCED_FACE('',(#456),#4083,.T.);
#4247=ADVANCED_FACE('',(#457),#4084,.T.);
#4248=ADVANCED_FACE('',(#458),#4085,.T.);
#4249=ADVANCED_FACE('',(#459),#71,.T.);
#4250=ADVANCED_FACE('',(#460),#274,.T.);
#4251=ADVANCED_FACE('',(#461),#4086,.T.);
#4252=ADVANCED_FACE('',(#462),#199,.F.);
#4253=ADVANCED_FACE('',(#463),#200,.F.);
#4254=ADVANCED_FACE('',(#464),#4087,.T.);
#4255=ADVANCED_FACE('',(#465),#72,.T.);
#4256=ADVANCED_FACE('',(#466),#4088,.T.);
#4257=ADVANCED_FACE('',(#467),#275,.T.);
#4258=ADVANCED_FACE('',(#468),#276,.T.);
#4259=ADVANCED_FACE('',(#469,#154),#201,.T.);
#4260=ADVANCED_FACE('',(#470),#90,.T.);
#4261=ADVANCED_FACE('',(#471),#73,.T.);
#4262=ADVANCED_FACE('',(#472),#4089,.T.);
#4263=ADVANCED_FACE('',(#473),#4090,.T.);
#4264=ADVANCED_FACE('',(#474),#74,.T.);
#4265=ADVANCED_FACE('',(#475),#202,.F.);
#4266=ADVANCED_FACE('',(#476),#4091,.T.);
#4267=ADVANCED_FACE('',(#477),#4092,.F.);
#4268=ADVANCED_FACE('',(#478),#314,.F.);
#4269=ADVANCED_FACE('',(#479),#4093,.T.);
#4270=ADVANCED_FACE('',(#480),#75,.T.);
#4271=ADVANCED_FACE('',(#481),#76,.T.);
#4272=ADVANCED_FACE('',(#482),#315,.F.);
#4273=ADVANCED_FACE('',(#483),#297,.T.);
#4274=ADVANCED_FACE('',(#484),#316,.F.);
#4275=ADVANCED_FACE('',(#485),#203,.F.);
#4276=ADVANCED_FACE('',(#486),#317,.F.);
#4277=ADVANCED_FACE('',(#487),#204,.F.);
#4278=ADVANCED_FACE('',(#488),#318,.F.);
#4279=ADVANCED_FACE('',(#489,#155),#205,.T.);
#4280=ADVANCED_FACE('',(#490),#91,.F.);
#4387=CLOSED_SHELL('',(#4228,#4229,#4230,#4231,#4232,#4233,#4234,#4235,
#4236,#4237,#4238,#4239,#4240,#4241,#4242,#4243,#4244,#4245,#4246,#4247,
#4248,#4249,#4250,#4251,#4252,#4253,#4254,#4255,#4256,#4257,#4258,#4259,
#4260,#4261,#4262,#4263,#4264,#4265,#4266,#4267,#4268,#4269,#4270,#4271,
#4272,#4273,#4274,#4275,#4276,#4277,#4278,#4279,#4280));
#4704=AXIS2_PLACEMENT_3D('',#10419,#5488,#5489);
#4705=AXIS2_PLACEMENT_3D('',#10420,#5490,#5491);
#4706=AXIS2_PLACEMENT_3D('',#10423,#5492,#5493);
#4707=AXIS2_PLACEMENT_3D('',#10425,#5494,#5495);
#4708=AXIS2_PLACEMENT_3D('',#10427,#5496,#5497);
#4709=AXIS2_PLACEMENT_3D('',#10428,#5498,#5499);
#4710=AXIS2_PLACEMENT_3D('',#10429,#5500,#5501);
#4711=AXIS2_PLACEMENT_3D('',#10436,#5502,#5503);
#4712=AXIS2_PLACEMENT_3D('',#10437,#5504,#5505);
#4713=AXIS2_PLACEMENT_3D('',#10444,#5506,#5507);
#4714=AXIS2_PLACEMENT_3D('',#10471,#5508,#5509);
#4715=AXIS2_PLACEMENT_3D('',#10476,#5510,#5511);
#4716=AXIS2_PLACEMENT_3D('',#10480,#5513,#5514);
#4717=AXIS2_PLACEMENT_3D('',#10482,#5516,#5517);
#4718=AXIS2_PLACEMENT_3D('',#10596,#5519,#5520);
#4719=AXIS2_PLACEMENT_3D('',#10620,#5521,#5522);
#4720=AXIS2_PLACEMENT_3D('',#10643,#5523,#5524);
#4721=AXIS2_PLACEMENT_3D('',#10645,#5525,#5526);
#4722=AXIS2_PLACEMENT_3D('',#10646,#5527,#5528);
#4723=AXIS2_PLACEMENT_3D('',#10647,#5529,#5530);
#4724=AXIS2_PLACEMENT_3D('',#10648,#5531,#5532);
#4725=AXIS2_PLACEMENT_3D('',#11006,#5533,#5534);
#4726=AXIS2_PLACEMENT_3D('',#11106,#5536,#5537);
#4727=AXIS2_PLACEMENT_3D('',#11135,#5538,#5539);
#4728=AXIS2_PLACEMENT_3D('',#11137,#5540,#5541);
#4729=AXIS2_PLACEMENT_3D('',#11139,#5543,#5544);
#4730=AXIS2_PLACEMENT_3D('',#11142,#5545,#5546);
#4731=AXIS2_PLACEMENT_3D('',#11143,#5547,#5548);
#4732=AXIS2_PLACEMENT_3D('',#11145,#5549,#5550);
#4733=AXIS2_PLACEMENT_3D('',#11146,#5551,#5552);
#4734=AXIS2_PLACEMENT_3D('',#11147,#5553,#5554);
#4735=AXIS2_PLACEMENT_3D('',#11152,#5556,#5557);
#4736=AXIS2_PLACEMENT_3D('',#11156,#5560,#5561);
#4737=AXIS2_PLACEMENT_3D('',#11158,#5562,#5563);
#4738=AXIS2_PLACEMENT_3D('',#11160,#5565,#5566);
#4739=AXIS2_PLACEMENT_3D('',#11162,#5567,#5568);
#4740=AXIS2_PLACEMENT_3D('',#11165,#5570,#5571);
#4741=AXIS2_PLACEMENT_3D('',#11166,#5572,#5573);
#4742=AXIS2_PLACEMENT_3D('',#11169,#5575,#5576);
#4743=AXIS2_PLACEMENT_3D('',#11170,#5577,#5578);
#4744=AXIS2_PLACEMENT_3D('',#11172,#5579,#5580);
#4745=AXIS2_PLACEMENT_3D('',#11173,#5581,#5582);
#4746=AXIS2_PLACEMENT_3D('',#11174,#5583,#5584);
#4747=AXIS2_PLACEMENT_3D('',#11176,#5585,#5586);
#4748=AXIS2_PLACEMENT_3D('',#11177,#5587,#5588);
#4749=AXIS2_PLACEMENT_3D('',#11178,#5589,#5590);
#4750=AXIS2_PLACEMENT_3D('',#11182,#5592,#5593);
#4751=AXIS2_PLACEMENT_3D('',#11184,#5595,#5596);
#4752=AXIS2_PLACEMENT_3D('',#11188,#5599,#5600);
#4753=AXIS2_PLACEMENT_3D('',#11192,#5603,#5604);
#4754=AXIS2_PLACEMENT_3D('',#11194,#5605,#5606);
#4755=AXIS2_PLACEMENT_3D('',#11197,#5608,#5609);
#4756=AXIS2_PLACEMENT_3D('',#11198,#5610,#5611);
#4757=AXIS2_PLACEMENT_3D('',#11200,#5612,#5613);
#4758=AXIS2_PLACEMENT_3D('',#11201,#5614,#5615);
#4759=AXIS2_PLACEMENT_3D('',#11202,#5616,#5617);
#4760=AXIS2_PLACEMENT_3D('',#11204,#5619,#5620);
#4761=AXIS2_PLACEMENT_3D('',#11206,#5621,#5622);
#4762=AXIS2_PLACEMENT_3D('',#11208,#5623,#5624);
#4763=AXIS2_PLACEMENT_3D('',#11209,#5625,#5626);
#4764=AXIS2_PLACEMENT_3D('',#11210,#5627,#5628);
#4765=AXIS2_PLACEMENT_3D('',#11212,#5629,#5630);
#4766=AXIS2_PLACEMENT_3D('',#11214,#5631,#5632);
#4767=AXIS2_PLACEMENT_3D('',#11216,#5633,#5634);
#4768=AXIS2_PLACEMENT_3D('',#11217,#5635,#5636);
#4769=AXIS2_PLACEMENT_3D('',#11218,#5637,#5638);
#4770=AXIS2_PLACEMENT_3D('',#11220,#5640,#5641);
#4771=AXIS2_PLACEMENT_3D('',#11224,#5643,#5644);
#4772=AXIS2_PLACEMENT_3D('',#11225,#5645,#5646);
#4773=AXIS2_PLACEMENT_3D('',#11226,#5647,#5648);
#4774=AXIS2_PLACEMENT_3D('',#11228,#5649,#5650);
#4775=AXIS2_PLACEMENT_3D('',#11229,#5651,#5652);
#4776=AXIS2_PLACEMENT_3D('',#11230,#5653,#5654);
#4777=AXIS2_PLACEMENT_3D('',#11232,#5656,#5657);
#4778=AXIS2_PLACEMENT_3D('',#11234,#5658,#5659);
#4779=AXIS2_PLACEMENT_3D('',#11237,#5662,#5663);
#4780=AXIS2_PLACEMENT_3D('',#11238,#5664,#5665);
#4781=AXIS2_PLACEMENT_3D('',#11239,#5666,#5667);
#4782=AXIS2_PLACEMENT_3D('',#11241,#5669,#5670);
#4783=AXIS2_PLACEMENT_3D('',#11242,#5671,#5672);
#4784=AXIS2_PLACEMENT_3D('',#11349,#5673,#5674);
#4785=AXIS2_PLACEMENT_3D('',#11372,#5675,#5676);
#4786=AXIS2_PLACEMENT_3D('',#11373,#5677,#5678);
#4787=AXIS2_PLACEMENT_3D('',#11376,#5680,#5681);
#4788=AXIS2_PLACEMENT_3D('',#11377,#5682,#5683);
#4789=AXIS2_PLACEMENT_3D('',#11378,#5684,#5685);
#4790=AXIS2_PLACEMENT_3D('',#11379,#5686,#5687);
#4791=AXIS2_PLACEMENT_3D('',#11380,#5688,#5689);
#4792=AXIS2_PLACEMENT_3D('',#11719,#5690,#5691);
#4793=AXIS2_PLACEMENT_3D('',#11751,#5693,#5694);
#4794=AXIS2_PLACEMENT_3D('',#11786,#5695,#5696);
#4795=AXIS2_PLACEMENT_3D('',#11787,#5697,#5698);
#5488=DIRECTION('axis',(0.,0.,1.));
#5489=DIRECTION('refdir',(1.,0.,0.));
#5490=DIRECTION('center_axis',(1.,0.,0.));
#5491=DIRECTION('ref_axis',(0.,-1.,1.83697019872103E-16));
#5492=DIRECTION('center_axis',(-1.5851531306331E-14,-0.044221029995557,
0.999021771787849));
#5493=DIRECTION('ref_axis',(-1.,-1.77635683940025E-14,-1.66533453693773E-14));
#5494=DIRECTION('center_axis',(1.,0.,0.));
#5495=DIRECTION('ref_axis',(0.,-1.,3.06161699786838E-17));
#5496=DIRECTION('center_axis',(2.43686520408589E-13,-0.0442210299954363,
-0.999021771787854));
#5497=DIRECTION('ref_axis',(-0.640184399668964,-0.767469783864776,0.0339715362478869));
#5498=DIRECTION('center_axis',(-1.,0.,0.));
#5499=DIRECTION('ref_axis',(0.,-1.,1.83697019872103E-16));
#5500=DIRECTION('center_axis',(-0.449113375415322,-0.210147679264594,-0.868409539861673));
#5501=DIRECTION('ref_axis',(-0.786560864598894,-0.368045017904336,0.495847628891413));
#5502=DIRECTION('center_axis',(0.,-1.,0.));
#5503=DIRECTION('ref_axis',(-0.707106781186548,0.,0.707106781186547));
#5504=DIRECTION('center_axis',(0.449113375415322,0.210147679264594,-0.868409539861672));
#5505=DIRECTION('ref_axis',(-0.786560864598894,-0.368045017904336,-0.495847628891415));
#5506=DIRECTION('center_axis',(0.,-1.,0.));
#5507=DIRECTION('ref_axis',(-0.707106781186548,0.,-0.707106781186547));
#5508=DIRECTION('center_axis',(0.767910450456811,-0.640557210621517,-3.00737669654705E-13));
#5509=DIRECTION('ref_axis',(-0.640184399664482,-0.76746351858997,-0.0341127844030622));
#5510=DIRECTION('center_axis',(0.,-1.,0.));
#5511=DIRECTION('ref_axis',(-0.707106781186548,0.,-0.707106781186547));
#5512=DIRECTION('',(0.,1.,0.));
#5513=DIRECTION('center_axis',(0.,-1.,0.));
#5514=DIRECTION('ref_axis',(-1.,0.,0.));
#5515=DIRECTION('',(0.,-1.,0.));
#5516=DIRECTION('center_axis',(-1.,0.,0.));
#5517=DIRECTION('ref_axis',(0.,0.,1.));
#5518=DIRECTION('',(0.,-1.,0.));
#5519=DIRECTION('center_axis',(6.37222258072231E-14,-0.0444048938881032,
-0.999013616222915));
#5520=DIRECTION('ref_axis',(-0.0166242555004783,-0.998875560049686,0.0443987574655116));
#5521=DIRECTION('center_axis',(2.56046860681907E-14,-0.0444048938880752,
0.999013616222917));
#5522=DIRECTION('ref_axis',(-0.640184399664478,-0.767463518589973,-0.0341127844030666));
#5523=DIRECTION('center_axis',(-0.953150734475215,0.258173802549692,-0.157638716838187));
#5524=DIRECTION('ref_axis',(-0.302495747688061,-0.813494243814166,0.496712631117691));
#5525=DIRECTION('center_axis',(-0.999861534547107,0.0166406650439521,0.));
#5526=DIRECTION('ref_axis',(-1.68476343986872E-13,3.5527136788006E-14,1.));
#5527=DIRECTION('center_axis',(0.76791045045681,-0.640557210621518,1.08864901799987E-13));
#5528=DIRECTION('ref_axis',(-1.68476343986872E-13,3.5527136788006E-14,1.));
#5529=DIRECTION('center_axis',(-0.953150734475031,0.258173802550189,0.15763871683849));
#5530=DIRECTION('ref_axis',(-0.302495747688635,-0.813494243814005,-0.496712631117605));
#5531=DIRECTION('center_axis',(-0.999861534547107,0.0166406650439596,0.));
#5532=DIRECTION('ref_axis',(-3.95794508278868E-13,-1.77635683940025E-14,
-1.));
#5533=DIRECTION('center_axis',(0.,0.,1.));
#5534=DIRECTION('ref_axis',(1.,0.,0.));
#5535=DIRECTION('',(0.,1.,0.));
#5536=DIRECTION('center_axis',(-7.51780949620696E-14,3.98534670278357E-13,
1.));
#5537=DIRECTION('ref_axis',(-0.987805559694749,-0.155692569624061,-1.22124532708767E-14));
#5538=DIRECTION('center_axis',(-1.,0.,0.));
#5539=DIRECTION('ref_axis',(0.,1.,0.));
#5540=DIRECTION('center_axis',(1.,0.,0.));
#5541=DIRECTION('ref_axis',(0.,0.,-1.));
#5542=DIRECTION('',(-0.196116135138184,-0.98058067569092,-1.20086498579063E-16));
#5543=DIRECTION('center_axis',(1.,0.,0.));
#5544=DIRECTION('ref_axis',(0.,0.,-1.));
#5545=DIRECTION('center_axis',(-1.,0.,0.));
#5546=DIRECTION('ref_axis',(0.,-1.,1.83697019872103E-16));
#5547=DIRECTION('center_axis',(-1.,0.,0.));
#5548=DIRECTION('ref_axis',(0.,-1.,1.83697019872103E-16));
#5549=DIRECTION('center_axis',(0.,-1.,-1.22464679914735E-16));
#5550=DIRECTION('ref_axis',(0.,-1.22464679914735E-16,1.));
#5551=DIRECTION('center_axis',(1.,0.,0.));
#5552=DIRECTION('ref_axis',(0.,-1.,1.83697019872103E-16));
#5553=DIRECTION('center_axis',(-1.,0.,0.));
#5554=DIRECTION('ref_axis',(0.,0.,1.));
#5555=DIRECTION('',(0.,1.,0.));
#5556=DIRECTION('center_axis',(-1.,0.,0.));
#5557=DIRECTION('ref_axis',(0.,-1.,1.83697019872103E-16));
#5558=DIRECTION('',(0.,-1.,0.));
#5559=DIRECTION('',(0.,0.,-1.));
#5560=DIRECTION('center_axis',(1.,0.,0.));
#5561=DIRECTION('ref_axis',(0.,1.,0.));
#5562=DIRECTION('center_axis',(1.,0.,0.));
#5563=DIRECTION('ref_axis',(0.,0.,-1.));
#5564=DIRECTION('',(-1.,0.,0.));
#5565=DIRECTION('center_axis',(0.,0.,1.));
#5566=DIRECTION('ref_axis',(-0.707106781186546,-0.707106781186549,0.));
#5567=DIRECTION('center_axis',(0.,-0.707106781186547,-0.707106781186548));
#5568=DIRECTION('ref_axis',(0.,-0.707106781186548,0.707106781186547));
#5569=DIRECTION('',(0.,0.,1.));
#5570=DIRECTION('center_axis',(0.,0.707106781186547,-0.707106781186548));
#5571=DIRECTION('ref_axis',(0.,-0.707106781186548,-0.707106781186547));
#5572=DIRECTION('center_axis',(0.,-1.,0.));
#5573=DIRECTION('ref_axis',(-0.707106781186548,0.,-0.707106781186547));
#5574=DIRECTION('',(0.,-1.,0.));
#5575=DIRECTION('center_axis',(0.,1.,0.));
#5576=DIRECTION('ref_axis',(0.,0.,-1.));
#5577=DIRECTION('center_axis',(0.288199153586547,-0.87432067514108,0.390518379711947));
#5578=DIRECTION('ref_axis',(-0.519169991490067,-0.485348696321363,-0.70349069852796));
#5579=DIRECTION('center_axis',(-1.,0.,0.));
#5580=DIRECTION('ref_axis',(0.,-0.567877810008977,-0.823112867655104));
#5581=DIRECTION('center_axis',(0.,0.355029585798816,-0.934855065348378));
#5582=DIRECTION('ref_axis',(0.,0.934855065348378,0.355029585798816));
#5583=DIRECTION('center_axis',(1.,0.,0.));
#5584=DIRECTION('ref_axis',(0.,-1.,1.83697019872103E-16));
#5585=DIRECTION('center_axis',(1.,0.,0.));
#5586=DIRECTION('ref_axis',(0.,-1.,1.83697019872103E-16));
#5587=DIRECTION('center_axis',(0.,0.355029585798817,0.934855065348378));
#5588=DIRECTION('ref_axis',(0.,-0.934855065348378,0.355029585798817));
#5589=DIRECTION('center_axis',(1.,0.,0.));
#5590=DIRECTION('ref_axis',(0.,-0.567877810008977,-0.823112867655104));
#5591=DIRECTION('',(1.,0.,0.));
#5592=DIRECTION('center_axis',(1.,0.,0.));
#5593=DIRECTION('ref_axis',(0.,-0.567877810008977,-0.823112867655104));
#5594=DIRECTION('',(-1.,0.,0.));
#5595=DIRECTION('center_axis',(0.,0.,1.));
#5596=DIRECTION('ref_axis',(1.,0.,0.));
#5597=DIRECTION('',(-1.,0.,0.));
#5598=DIRECTION('',(0.,1.,0.));
#5599=DIRECTION('center_axis',(0.,1.,0.));
#5600=DIRECTION('ref_axis',(-1.,0.,0.));
#5601=DIRECTION('',(1.,0.,0.));
#5602=DIRECTION('',(0.,0.,-1.));
#5603=DIRECTION('center_axis',(0.,0.,-1.));
#5604=DIRECTION('ref_axis',(0.707106781186544,-0.707106781186551,0.));
#5605=DIRECTION('center_axis',(0.,-0.707106781186549,-0.707106781186546));
#5606=DIRECTION('ref_axis',(-4.90653893338679E-17,-0.707106781186546,0.707106781186549));
#5607=DIRECTION('',(0.,0.,1.));
#5608=DIRECTION('center_axis',(0.,0.707106781186547,-0.707106781186548));
#5609=DIRECTION('ref_axis',(0.,0.707106781186548,0.707106781186547));
#5610=DIRECTION('center_axis',(-0.288199153586547,-0.87432067514108,0.390518379711947));
#5611=DIRECTION('ref_axis',(0.519169991490067,-0.485348696321362,-0.703490698527961));
#5612=DIRECTION('center_axis',(0.,-1.,-2.22044604925031E-15));
#5613=DIRECTION('ref_axis',(0.,2.22044604925031E-15,-1.));
#5614=DIRECTION('center_axis',(0.,0.355029585798817,-0.934855065348378));
#5615=DIRECTION('ref_axis',(0.,0.934855065348378,0.355029585798817));
#5616=DIRECTION('center_axis',(0.,1.,0.));
#5617=DIRECTION('ref_axis',(0.707106781186547,0.,-0.707106781186548));
#5618=DIRECTION('',(0.,-1.,0.));
#5619=DIRECTION('center_axis',(1.,0.,0.));
#5620=DIRECTION('ref_axis',(0.,-1.,1.83697019872103E-16));
#5621=DIRECTION('center_axis',(1.,0.,0.));
#5622=DIRECTION('ref_axis',(0.,-0.999438109969484,0.0335181195866625));
#5623=DIRECTION('center_axis',(1.28747119532049E-15,-0.355029585798816,
-0.934855065348379));
#5624=DIRECTION('ref_axis',(1.,-2.22044604925031E-15,2.22044604925031E-15));
#5625=DIRECTION('center_axis',(-1.,0.,0.));
#5626=DIRECTION('ref_axis',(0.,-0.999438109969484,0.0335181195866626));
#5627=DIRECTION('center_axis',(1.,0.,0.));
#5628=DIRECTION('ref_axis',(0.,0.,-1.));
#5629=DIRECTION('center_axis',(-1.,0.,0.));
#5630=DIRECTION('ref_axis',(0.,-1.,1.83697019872103E-16));
#5631=DIRECTION('center_axis',(0.,-1.,-1.22464679914735E-16));
#5632=DIRECTION('ref_axis',(0.,-1.22464679914735E-16,1.));
#5633=DIRECTION('center_axis',(1.,0.,0.));
#5634=DIRECTION('ref_axis',(0.,-1.,3.06161699786838E-17));
#5635=DIRECTION('center_axis',(1.,0.,0.));
#5636=DIRECTION('ref_axis',(0.,-1.,3.06161699786838E-17));
#5637=DIRECTION('center_axis',(1.,0.,0.));
#5638=DIRECTION('ref_axis',(0.,0.,-1.));
#5639=DIRECTION('',(0.,1.,0.));
#5640=DIRECTION('center_axis',(-1.,0.,0.));
#5641=DIRECTION('ref_axis',(0.,1.,0.));
#5642=DIRECTION('',(-0.171609399198264,-0.985165069471513,-1.20647924896007E-16));
#5643=DIRECTION('center_axis',(1.,0.,0.));
#5644=DIRECTION('ref_axis',(0.,0.,-1.));
#5645=DIRECTION('center_axis',(1.,0.,0.));
#5646=DIRECTION('ref_axis',(0.,0.,-1.));
#5647=DIRECTION('center_axis',(0.288199153586548,-0.874320675141079,-0.390518379711948));
#5648=DIRECTION('ref_axis',(-0.519169991490068,-0.485348696321364,0.703490698527959));
#5649=DIRECTION('center_axis',(-1.,0.,0.));
#5650=DIRECTION('ref_axis',(0.,0.,1.));
#5651=DIRECTION('center_axis',(0.,-1.,0.));
#5652=DIRECTION('ref_axis',(-1.,0.,0.));
#5653=DIRECTION('center_axis',(0.,1.,0.));
#5654=DIRECTION('ref_axis',(-0.707106781186548,0.,0.707106781186547));
#5655=DIRECTION('',(0.,1.,0.));
#5656=DIRECTION('center_axis',(-1.,0.,0.));
#5657=DIRECTION('ref_axis',(0.,-0.567877810008977,0.823112867655104));
#5658=DIRECTION('center_axis',(-1.,0.,0.));
#5659=DIRECTION('ref_axis',(0.,-0.934855065348378,0.355029585798817));
#5660=DIRECTION('',(-1.,0.,0.));
#5661=DIRECTION('',(1.,0.,0.));
#5662=DIRECTION('center_axis',(-0.288199153586547,-0.87432067514108,-0.390518379711947));
#5663=DIRECTION('ref_axis',(0.519169991490067,-0.485348696321363,0.70349069852796));
#5664=DIRECTION('center_axis',(0.,-1.,0.));
#5665=DIRECTION('ref_axis',(0.707106781186546,0.,0.707106781186549));
#5666=DIRECTION('center_axis',(0.,0.,-1.));
#5667=DIRECTION('ref_axis',(-1.,0.,0.));
#5668=DIRECTION('',(0.,-1.,0.));
#5669=DIRECTION('center_axis',(0.,-1.,0.));
#5670=DIRECTION('ref_axis',(0.707106781186547,0.,0.707106781186548));
#5671=DIRECTION('center_axis',(1.,0.,0.));
#5672=DIRECTION('ref_axis',(0.,-1.,1.22464679914735E-16));
#5673=DIRECTION('center_axis',(0.,-0.043896042544273,-0.999036104176897));
#5674=DIRECTION('ref_axis',(-1.,0.,0.));
#5675=DIRECTION('center_axis',(0.,-0.0438960425442462,0.999036104176898));
#5676=DIRECTION('ref_axis',(-0.321450532286738,0.946013634312855,0.0415663203417933));
#5677=DIRECTION('center_axis',(0.,1.,0.));
#5678=DIRECTION('ref_axis',(-0.707106781186548,0.,0.707106781186547));
#5679=DIRECTION('',(0.,1.,0.));
#5680=DIRECTION('center_axis',(0.,-1.,0.));
#5681=DIRECTION('ref_axis',(4.7642445544227E-13,0.,1.));
#5682=DIRECTION('center_axis',(-0.413050977203529,0.295699193086847,-0.861365704819386));
#5683=DIRECTION('ref_axis',(-0.700390161752567,0.501402531664142,0.507985356640329));
#5684=DIRECTION('center_axis',(-0.946831936616679,-0.321728587170473,0.));
#5685=DIRECTION('ref_axis',(-3.02535774210343E-14,-1.77635683940018E-14,
1.));
#5686=DIRECTION('center_axis',(0.413050977203297,-0.295699193086435,-0.861365704819639));
#5687=DIRECTION('ref_axis',(-0.700390161752968,0.501402531664014,-0.507985356639902));
#5688=DIRECTION('center_axis',(-0.946831936616687,-0.321728587170451,0.));
#5689=DIRECTION('ref_axis',(1.69586567011493E-13,8.88178419700125E-14,-1.));
#5690=DIRECTION('center_axis',(0.,0.,-1.));
#5691=DIRECTION('ref_axis',(-1.,0.,0.));
#5692=DIRECTION('',(0.,-1.,0.));
#5693=DIRECTION('center_axis',(1.,0.,0.));
#5694=DIRECTION('ref_axis',(0.,1.,0.));
#5695=DIRECTION('center_axis',(-1.,0.,0.));
#5696=DIRECTION('ref_axis',(0.,0.,1.));
#5697=DIRECTION('center_axis',(-1.,0.,0.));
#5698=DIRECTION('ref_axis',(0.,-1.,1.22464679914735E-16));
#10419=CARTESIAN_POINT('',(0.,0.,0.));
#10420=CARTESIAN_POINT('Origin',(0.5,0.,0.));
#10421=CARTESIAN_POINT('',(0.,56.4788841358559,2.5));
#10422=CARTESIAN_POINT('',(0.179907800166174,56.0951492439243,2.48301423187597));
#10423=CARTESIAN_POINT('Origin',(0.5,56.4788841358559,2.50000000000001));
#10424=CARTESIAN_POINT('',(0.17990780016617,56.0951492439243,-2.48301423187597));
#10425=CARTESIAN_POINT('Origin',(0.17990780016776,0.,-8.59550148320605E-15));
#10426=CARTESIAN_POINT('',(0.,56.4788841358559,-2.5));
#10427=CARTESIAN_POINT('Origin',(0.5,56.4788841358559,-2.49999999999988));
#10428=CARTESIAN_POINT('Origin',(0.,0.,0.));
#10429=CARTESIAN_POINT('Origin',(0.5,56.4788841358559,-2.5));
#10430=CARTESIAN_POINT('',(0.499999999997957,56.4788841358593,-2.));
#10431=CARTESIAN_POINT('Ctrl Pts',(0.179907800164864,56.095149243924,-2.48301423187597));
#10432=CARTESIAN_POINT('Ctrl Pts',(0.182694641762887,56.0984901824412,-2.3550199649901));
#10433=CARTESIAN_POINT('Ctrl Pts',(0.254541365578152,56.1846219120289,-2.1035560356539));
#10434=CARTESIAN_POINT('Ctrl Pts',(0.417965393799912,56.380538906701,-2.));
#10435=CARTESIAN_POINT('Ctrl Pts',(0.499999999997104,56.4788841358583,-2.));
#10436=CARTESIAN_POINT('Origin',(0.5,56.4788841358559,-2.5));
#10437=CARTESIAN_POINT('Origin',(0.5,56.4788841358559,2.5));
#10438=CARTESIAN_POINT('',(0.499999999997957,56.4788841358593,2.));
#10439=CARTESIAN_POINT('Ctrl Pts',(0.499999999997116,56.4788841358583,2.));
#10440=CARTESIAN_POINT('Ctrl Pts',(0.417965393799925,56.380538906701,2.));
#10441=CARTESIAN_POINT('Ctrl Pts',(0.254541365578165,56.1846219120289,2.1035560356539));
#10442=CARTESIAN_POINT('Ctrl Pts',(0.1826946417629,56.0984901824412,2.3550199649901));
#10443=CARTESIAN_POINT('Ctrl Pts',(0.179907800164876,56.095149243924,2.48301423187597));
#10444=CARTESIAN_POINT('Origin',(0.5,56.4788841358559,2.5));
#10445=CARTESIAN_POINT('Ctrl Pts',(0.499999999997116,56.4788841358583,2.));
#10446=CARTESIAN_POINT('Ctrl Pts',(0.593634842898508,56.4007786951615,2.));
#10447=CARTESIAN_POINT('Ctrl Pts',(0.687269529957182,56.3226730676369,2.));
#10448=CARTESIAN_POINT('Ctrl Pts',(0.780904059217746,56.2445672509427,2.));
#10449=CARTESIAN_POINT('Ctrl Pts',(0.417965393799925,56.380538906701,2.));
#10450=CARTESIAN_POINT('Ctrl Pts',(0.511602632292953,56.3024366043021,2.00000011921147));
#10451=CARTESIAN_POINT('Ctrl Pts',(0.605239657990774,56.2243340470848,1.99999987982881));
#10452=CARTESIAN_POINT('Ctrl Pts',(0.698876602273683,56.1462313952731,2.));
#10453=CARTESIAN_POINT('Ctrl Pts',(0.254541365578165,56.1846219120289,2.1035560356539));
#10454=CARTESIAN_POINT('Ctrl Pts',(0.348183189883171,56.1065256357554,2.10354935262451));
#10455=CARTESIAN_POINT('Ctrl Pts',(0.441824994766503,56.0284293435913,2.10354276030279));
#10456=CARTESIAN_POINT('Ctrl Pts',(0.53546656209897,55.9503327690787,2.1035360223157));
#10457=CARTESIAN_POINT('Ctrl Pts',(0.1826946417629,56.0984901824412,2.3550199649901));
#10458=CARTESIAN_POINT('Ctrl Pts',(0.276333332478559,56.0203903852816,2.35500062661495));
#10459=CARTESIAN_POINT('Ctrl Pts',(0.369971635899614,55.9422901242085,2.35498122632127));
#10460=CARTESIAN_POINT('Ctrl Pts',(0.463610044339371,55.8641900014912,2.35496172772305));
#10461=CARTESIAN_POINT('Ctrl Pts',(0.179907800164876,56.095149243924,2.48301423187597));
#10462=CARTESIAN_POINT('Ctrl Pts',(0.273542643066269,56.0170448409568,2.4829907879535));
#10463=CARTESIAN_POINT('Ctrl Pts',(0.367177330124943,55.9389402576093,2.48296724699913));
#10464=CARTESIAN_POINT('Ctrl Pts',(0.460811859385507,55.8608354916477,2.48294360779847));
#10465=CARTESIAN_POINT('',(0.780904059217604,56.2445672509427,2.));
#10466=CARTESIAN_POINT('Ctrl Pts',(0.499999999997116,56.4788841358583,2.));
#10467=CARTESIAN_POINT('Ctrl Pts',(0.593634842898508,56.4007786951615,2.));
#10468=CARTESIAN_POINT('Ctrl Pts',(0.687269529957182,56.3226730676369,2.));
#10469=CARTESIAN_POINT('Ctrl Pts',(0.780904059217746,56.2445672509427,2.));
#10470=CARTESIAN_POINT('',(0.460811859385445,55.8608354916477,2.48294360779849));
#10471=CARTESIAN_POINT('Origin',(0.7809040592178,56.2445672509427,2.5));
#10472=CARTESIAN_POINT('Ctrl Pts',(0.460811859385507,55.8608354916477,2.48294360779847));
#10473=CARTESIAN_POINT('Ctrl Pts',(0.367177330124943,55.9389402576093,2.48296724699913));
#10474=CARTESIAN_POINT('Ctrl Pts',(0.273542643066269,56.0170448409568,2.4829907879535));
#10475=CARTESIAN_POINT('Ctrl Pts',(0.179907800164876,56.095149243924,2.48301423187597));
#10476=CARTESIAN_POINT('Origin',(0.5,57.025,2.5));
#10477=CARTESIAN_POINT('',(0.,56.8978458123627,2.5));
#10478=CARTESIAN_POINT('',(0.,57.025,2.5));
#10479=CARTESIAN_POINT('',(0.500000000000237,56.8978458123627,2.));
#10480=CARTESIAN_POINT('Origin',(0.5,56.8978458123627,2.5));
#10481=CARTESIAN_POINT('',(0.5,57.025,2.));
#10482=CARTESIAN_POINT('Origin',(0.,57.3,0.));
#10483=CARTESIAN_POINT('',(0.,56.8978458123625,-2.49999999999977));
#10484=CARTESIAN_POINT('',(0.,57.025,-2.5));
#10485=CARTESIAN_POINT('Ctrl Pts',(0.,56.8978458123625,2.49999999999978));
#10486=CARTESIAN_POINT('Ctrl Pts',(0.,56.5290913566253,10.8925336660656));
#10487=CARTESIAN_POINT('Ctrl Pts',(0.,52.0239399392849,27.5104427981014));
#10488=CARTESIAN_POINT('Ctrl Pts',(0.,37.0895128901808,44.9505513524534));
#10489=CARTESIAN_POINT('Ctrl Pts',(0.,19.6413066333793,54.3407718417784));
#10490=CARTESIAN_POINT('Ctrl Pts',(0.,2.98972976337264,57.7126473424414));
#10491=CARTESIAN_POINT('Ctrl Pts',(0.,-13.9100795010715,56.0762889490297));
#10492=CARTESIAN_POINT('Ctrl Pts',(0.,-34.8726547481504,47.4775611101652));
#10493=CARTESIAN_POINT('Ctrl Pts',(0.,-48.6578954952714,32.3601597542925));
#10494=CARTESIAN_POINT('Ctrl Pts',(0.,-54.6754985459398,16.615078371656));
#10495=CARTESIAN_POINT('Ctrl Pts',(0.,-58.4322800872165,0.182637285551057));
#10496=CARTESIAN_POINT('Ctrl Pts',(0.,-55.3972091422166,-20.0478023034309));
#10497=CARTESIAN_POINT('Ctrl Pts',(0.,-42.7587268357465,-38.8566003856648));
#10498=CARTESIAN_POINT('Ctrl Pts',(0.,-29.6277979733952,-49.6176180623964));
#10499=CARTESIAN_POINT('Ctrl Pts',(0.,-13.9134722149986,-56.083084294608));
#10500=CARTESIAN_POINT('Ctrl Pts',(0.,2.99163137042858,-57.710045079662));
#10501=CARTESIAN_POINT('Ctrl Pts',(0.,19.6409629692718,-54.3421091676748));
#10502=CARTESIAN_POINT('Ctrl Pts',(0.,37.0902013849514,-44.9493511994273));
#10503=CARTESIAN_POINT('Ctrl Pts',(0.,52.0238383479187,-27.5106172571882));
#10504=CARTESIAN_POINT('Ctrl Pts',(0.,56.5290913566252,-10.8925336660656));
#10505=CARTESIAN_POINT('Ctrl Pts',(0.,56.8978458123625,-2.49999999999977));
#10506=CARTESIAN_POINT('Ctrl Pts',(0.772591931467417,55.7451294709179,2.47780062126729));
#10507=CARTESIAN_POINT('Ctrl Pts',(0.772591931467417,55.379709551606,10.6989547118962));
#10508=CARTESIAN_POINT('Ctrl Pts',(0.772591931467379,50.9581493156086,26.9764013787265));
#10509=CARTESIAN_POINT('Ctrl Pts',(0.772591931467366,36.3233521724092,44.0527896931361));
#10510=CARTESIAN_POINT('Ctrl Pts',(0.77259193146737,19.2256187449638,53.2486164943009));
#10511=CARTESIAN_POINT('Ctrl Pts',(0.772591931467382,2.91685365030647,56.5415921245837));
#10512=CARTESIAN_POINT('Ctrl Pts',(0.772591931467353,-13.6471652991449,
54.9460594777695));
#10513=CARTESIAN_POINT('Ctrl Pts',(0.77259193146742,-29.0305558907579,48.6064856663137));
#10514=CARTESIAN_POINT('Ctrl Pts',(0.772591931467399,-41.9074799864638,
38.0671554541429));
#10515=CARTESIAN_POINT('Ctrl Pts',(0.772591931467406,-51.1637806560337,
24.240464632067));
#10516=CARTESIAN_POINT('Ctrl Pts',(0.772591931467356,-56.0014365376947,
8.31948037804371));
#10517=CARTESIAN_POINT('Ctrl Pts',(0.772591931467423,-56.0009380440498,
-8.31968241557478));
#10518=CARTESIAN_POINT('Ctrl Pts',(0.772591931467387,-51.1640653905075,
-24.2409304612857));
#10519=CARTESIAN_POINT('Ctrl Pts',(0.772591931467385,-41.9071399938438,
-38.0674064524271));
#10520=CARTESIAN_POINT('Ctrl Pts',(0.772591931467373,-29.0304426638128,
-48.6065966625385));
#10521=CARTESIAN_POINT('Ctrl Pts',(0.772591931467365,-13.6468152705721,
-54.9457263658574));
#10522=CARTESIAN_POINT('Ctrl Pts',(0.772591931467323,2.91739716720752,-56.5422576232864));
#10523=CARTESIAN_POINT('Ctrl Pts',(0.772591931467349,19.2260068136787,-53.2483487259477));
#10524=CARTESIAN_POINT('Ctrl Pts',(0.772591931467411,36.3234077815813,-44.0527282308743));
#10525=CARTESIAN_POINT('Ctrl Pts',(0.772591931467395,50.9584317787812,-26.975898664924));
#10526=CARTESIAN_POINT('Ctrl Pts',(0.772591931467383,55.379709551606,-10.6989547118962));
#10527=CARTESIAN_POINT('Ctrl Pts',(0.772591931467384,55.7451294709179,-2.47780062126731));
#10528=CARTESIAN_POINT('Ctrl Pts',(0.659588674014702,55.747006472314,2.47788405160945));
#10529=CARTESIAN_POINT('Ctrl Pts',(0.659588674014702,55.3815762057712,10.6992709324469));
#10530=CARTESIAN_POINT('Ctrl Pts',(0.659588674014685,50.9598613650699,26.9773401036556));
#10531=CARTESIAN_POINT('Ctrl Pts',(0.659588674014669,36.3245761421025,44.0542605993868));
#10532=CARTESIAN_POINT('Ctrl Pts',(0.65958867401467,19.2262615067636,53.2504137911799));
#10533=CARTESIAN_POINT('Ctrl Pts',(0.659588674014682,2.91695282870238,56.543493263952));
#10534=CARTESIAN_POINT('Ctrl Pts',(0.659588674014657,-13.647622959522,54.9479091625884));
#10535=CARTESIAN_POINT('Ctrl Pts',(0.659588674014704,-29.0315351701335,
48.6081203793897));
#10536=CARTESIAN_POINT('Ctrl Pts',(0.659588674014695,-41.9088877796823,
38.0684377192795));
#10537=CARTESIAN_POINT('Ctrl Pts',(0.659588674014705,-51.1655032091182,
24.241282493667));
#10538=CARTESIAN_POINT('Ctrl Pts',(0.65958867401464,-56.0033201731021,8.31975571353977));
#10539=CARTESIAN_POINT('Ctrl Pts',(0.659588674014727,-56.0028236846315,
-8.31996139839591));
#10540=CARTESIAN_POINT('Ctrl Pts',(0.659588674014686,-51.1657866585822,
-24.2417444733812));
#10541=CARTESIAN_POINT('Ctrl Pts',(0.659588674014683,-41.9085495140753,
-38.0686899407466));
#10542=CARTESIAN_POINT('Ctrl Pts',(0.659588674014673,-29.0314210013225,
-48.608229623483));
#10543=CARTESIAN_POINT('Ctrl Pts',(0.659588674014657,-13.6472763990038,
-54.9475778572917));
#10544=CARTESIAN_POINT('Ctrl Pts',(0.659588674014636,2.91749931213322,-56.5441560813714));
#10545=CARTESIAN_POINT('Ctrl Pts',(0.659588674014654,19.2266538416122,-53.2501458099667));
#10546=CARTESIAN_POINT('Ctrl Pts',(0.659588674014694,36.3246254700402,-44.0542012209058));
#10547=CARTESIAN_POINT('Ctrl Pts',(0.659588674014703,50.960147755993,-26.9768360225067));
#10548=CARTESIAN_POINT('Ctrl Pts',(0.659588674014674,55.3815762057712,-10.6992709324469));
#10549=CARTESIAN_POINT('Ctrl Pts',(0.659588674014674,55.747006472314,-2.47788405160947));
#10550=CARTESIAN_POINT('Ctrl Pts',(0.547635364780324,55.788553938233,2.47973078401178));
#10551=CARTESIAN_POINT('Ctrl Pts',(0.547635364780324,55.4228512437384,10.7072467017526));
#10552=CARTESIAN_POINT('Ctrl Pts',(0.547635364780334,50.9978411885347,26.9974447290012));
#10553=CARTESIAN_POINT('Ctrl Pts',(0.547635364780309,36.3516483050864,44.0870941184864));
#10554=CARTESIAN_POINT('Ctrl Pts',(0.547635364780313,19.2405907536628,53.2901004080723));
#10555=CARTESIAN_POINT('Ctrl Pts',(0.547635364780321,2.91912675454844,56.5856344470053));
#10556=CARTESIAN_POINT('Ctrl Pts',(0.547635364780301,-13.6577944162708,
54.9888610887901));
#10557=CARTESIAN_POINT('Ctrl Pts',(0.547635364780325,-29.0531718969856,
48.6443474096255));
#10558=CARTESIAN_POINT('Ctrl Pts',(0.54763536478033,-41.9401220193493,38.0968095746887));
#10559=CARTESIAN_POINT('Ctrl Pts',(0.547635364780343,-51.2036361521209,
24.2593491172253));
#10560=CARTESIAN_POINT('Ctrl Pts',(0.547635364780263,-56.045058745482,8.32595650201345));
#10561=CARTESIAN_POINT('Ctrl Pts',(0.547635364780371,-56.044561806521,-8.32616219528814));
#10562=CARTESIAN_POINT('Ctrl Pts',(0.547635364780327,-51.2039198643548,
-24.2598115950628));
#10563=CARTESIAN_POINT('Ctrl Pts',(0.54763536478032,-41.9397834324552,-38.0970619357924));
#10564=CARTESIAN_POINT('Ctrl Pts',(0.547635364780315,-29.0530576804163,
-48.6444568050123));
#10565=CARTESIAN_POINT('Ctrl Pts',(0.547635364780284,-13.6574474589847,
-54.9885294642351));
#10566=CARTESIAN_POINT('Ctrl Pts',(0.547635364780292,2.91967352794025,-56.5862978660074));
#10567=CARTESIAN_POINT('Ctrl Pts',(0.547635364780297,19.2409832116612,-53.2898322352485));
#10568=CARTESIAN_POINT('Ctrl Pts',(0.547635364780317,36.3516979198253,-44.0870346127446));
#10569=CARTESIAN_POINT('Ctrl Pts',(0.547635364780352,50.9981276369736,-26.9969403259078));
#10570=CARTESIAN_POINT('Ctrl Pts',(0.547635364780302,55.4228512437384,-10.7072467017526));
#10571=CARTESIAN_POINT('Ctrl Pts',(0.547635364780302,55.788553938233,-2.4797307840118));
#10572=CARTESIAN_POINT('Ctrl Pts',(0.460811859385443,55.8608354916477,2.48294360779849));
#10573=CARTESIAN_POINT('Ctrl Pts',(0.460811859385443,55.4946570973774,10.7211617367507));
#10574=CARTESIAN_POINT('Ctrl Pts',(0.460811859385469,51.0639193575303,27.0323942894394));
#10575=CARTESIAN_POINT('Ctrl Pts',(0.46081185938544,36.3987458539618,44.1442267934859));
#10576=CARTESIAN_POINT('Ctrl Pts',(0.460811859385444,19.2655239324154,53.3591406886548));
#10577=CARTESIAN_POINT('Ctrl Pts',(0.46081185938545,2.92290794656755,56.6589513036287));
#10578=CARTESIAN_POINT('Ctrl Pts',(0.460811859385435,-13.6754917055233,
55.0601069283235));
#10579=CARTESIAN_POINT('Ctrl Pts',(0.460811859385444,-29.09081245727,48.7073745348389));
#10580=CARTESIAN_POINT('Ctrl Pts',(0.460811859385456,-41.9944642269539,
38.1461686185199));
#10581=CARTESIAN_POINT('Ctrl Pts',(0.460811859385471,-51.2699775116405,
24.290778762285));
#10582=CARTESIAN_POINT('Ctrl Pts',(0.460811859385381,-56.1176745559473,
8.33674850493155));
#10583=CARTESIAN_POINT('Ctrl Pts',(0.460811859385504,-56.1171750276162,
-8.33695096181688));
#10584=CARTESIAN_POINT('Ctrl Pts',(0.460811859385457,-51.2702628371164,
-24.2912455583908));
#10585=CARTESIAN_POINT('Ctrl Pts',(0.460811859385448,-41.9941235286365,
-38.1464201377825));
#10586=CARTESIAN_POINT('Ctrl Pts',(0.460811859385444,-29.0906989953083,
-48.7074857614504));
#10587=CARTESIAN_POINT('Ctrl Pts',(0.460811859385409,-13.6751409504222,
-55.0597731249957));
#10588=CARTESIAN_POINT('Ctrl Pts',(0.460811859385431,2.92345259160619,-56.6596181836576));
#10589=CARTESIAN_POINT('Ctrl Pts',(0.46081185938543,19.2659128066157,-53.3588723645147));
#10590=CARTESIAN_POINT('Ctrl Pts',(0.460811859385435,36.3988015785576,-44.1441652036514));
#10591=CARTESIAN_POINT('Ctrl Pts',(0.460811859385486,51.0642024069907,-27.0318905321913));
#10592=CARTESIAN_POINT('Ctrl Pts',(0.460811859385425,55.4946570973774,-10.7211617367508));
#10593=CARTESIAN_POINT('Ctrl Pts',(0.460811859385425,55.8608354916477,-2.48294360779851));
#10594=CARTESIAN_POINT('',(0.772591931467425,55.7451294709179,-2.47780062126728));
#10595=CARTESIAN_POINT('',(0.460811859385434,55.8608354916477,-2.48294360779851));
#10596=CARTESIAN_POINT('Origin',(0.780904059217663,56.2445672509427,-2.50000000000004));
#10597=CARTESIAN_POINT('Ctrl Pts',(0.460811859385425,55.8608354916477,-2.48294360779851));
#10598=CARTESIAN_POINT('Ctrl Pts',(0.460811859385425,55.4946570973774,-10.7211617367508));
#10599=CARTESIAN_POINT('Ctrl Pts',(0.460811859385486,51.0642024069907,-27.0318905321913));
#10600=CARTESIAN_POINT('Ctrl Pts',(0.460811859385435,36.3988015785576,-44.1441652036514));
#10601=CARTESIAN_POINT('Ctrl Pts',(0.46081185938543,19.2659128066157,-53.3588723645147));
#10602=CARTESIAN_POINT('Ctrl Pts',(0.460811859385431,2.92345259160619,-56.6596181836576));
#10603=CARTESIAN_POINT('Ctrl Pts',(0.460811859385409,-13.6751409504222,
-55.0597731249957));
#10604=CARTESIAN_POINT('Ctrl Pts',(0.460811859385444,-29.0906989953083,
-48.7074857614504));
#10605=CARTESIAN_POINT('Ctrl Pts',(0.460811859385448,-41.9941235286365,
-38.1464201377825));
#10606=CARTESIAN_POINT('Ctrl Pts',(0.460811859385457,-51.2702628371164,
-24.2912455583908));
#10607=CARTESIAN_POINT('Ctrl Pts',(0.460811859385504,-56.1171750276162,
-8.33695096181688));
#10608=CARTESIAN_POINT('Ctrl Pts',(0.460811859385381,-56.1176745559473,
8.33674850493155));
#10609=CARTESIAN_POINT('Ctrl Pts',(0.460811859385471,-51.2699775116405,
24.290778762285));
#10610=CARTESIAN_POINT('Ctrl Pts',(0.460811859385456,-41.9944642269539,
38.1461686185199));
#10611=CARTESIAN_POINT('Ctrl Pts',(0.460811859385444,-29.09081245727,48.7073745348389));
#10612=CARTESIAN_POINT('Ctrl Pts',(0.460811859385435,-13.6754917055233,
55.0601069283235));
#10613=CARTESIAN_POINT('Ctrl Pts',(0.46081185938545,2.92290794656755,56.6589513036287));
#10614=CARTESIAN_POINT('Ctrl Pts',(0.460811859385444,19.2655239324154,53.3591406886548));
#10615=CARTESIAN_POINT('Ctrl Pts',(0.46081185938544,36.3987458539618,44.1442267934859));
#10616=CARTESIAN_POINT('Ctrl Pts',(0.460811859385469,51.0639193575303,27.0323942894394));
#10617=CARTESIAN_POINT('Ctrl Pts',(0.460811859385443,55.4946570973774,10.7211617367507));
#10618=CARTESIAN_POINT('Ctrl Pts',(0.460811859385443,55.8608354916477,2.48294360779849));
#10619=CARTESIAN_POINT('',(0.772591931467348,55.7451294709179,2.47780062126728));
#10620=CARTESIAN_POINT('Origin',(0.780904059217683,56.2445672509427,2.50000000000002));
#10621=CARTESIAN_POINT('Ctrl Pts',(0.772591931467417,55.7451294709179,2.47780062126729));
#10622=CARTESIAN_POINT('Ctrl Pts',(0.772591931467417,55.379709551606,10.6989547118962));
#10623=CARTESIAN_POINT('Ctrl Pts',(0.772591931467379,50.9581493156086,26.9764013787265));
#10624=CARTESIAN_POINT('Ctrl Pts',(0.772591931467366,36.3233521724092,44.0527896931361));
#10625=CARTESIAN_POINT('Ctrl Pts',(0.77259193146737,19.2256187449638,53.2486164943009));
#10626=CARTESIAN_POINT('Ctrl Pts',(0.772591931467382,2.91685365030647,56.5415921245837));
#10627=CARTESIAN_POINT('Ctrl Pts',(0.772591931467353,-13.6471652991449,
54.9460594777695));
#10628=CARTESIAN_POINT('Ctrl Pts',(0.77259193146742,-29.0305558907579,48.6064856663137));
#10629=CARTESIAN_POINT('Ctrl Pts',(0.772591931467399,-41.9074799864638,
38.0671554541429));
#10630=CARTESIAN_POINT('Ctrl Pts',(0.772591931467406,-51.1637806560337,
24.240464632067));
#10631=CARTESIAN_POINT('Ctrl Pts',(0.772591931467356,-56.0014365376947,
8.31948037804371));
#10632=CARTESIAN_POINT('Ctrl Pts',(0.772591931467423,-56.0009380440498,
-8.31968241557478));
#10633=CARTESIAN_POINT('Ctrl Pts',(0.772591931467387,-51.1640653905075,
-24.2409304612857));
#10634=CARTESIAN_POINT('Ctrl Pts',(0.772591931467385,-41.9071399938438,
-38.0674064524271));
#10635=CARTESIAN_POINT('Ctrl Pts',(0.772591931467373,-29.0304426638128,
-48.6065966625385));
#10636=CARTESIAN_POINT('Ctrl Pts',(0.772591931467365,-13.6468152705721,
-54.9457263658574));
#10637=CARTESIAN_POINT('Ctrl Pts',(0.772591931467323,2.91739716720752,-56.5422576232864));
#10638=CARTESIAN_POINT('Ctrl Pts',(0.772591931467349,19.2260068136787,-53.2483487259477));
#10639=CARTESIAN_POINT('Ctrl Pts',(0.772591931467411,36.3234077815813,-44.0527282308743));
#10640=CARTESIAN_POINT('Ctrl Pts',(0.772591931467395,50.9584317787812,-26.975898664924));
#10641=CARTESIAN_POINT('Ctrl Pts',(0.772591931467383,55.379709551606,-10.6989547118962));
#10642=CARTESIAN_POINT('Ctrl Pts',(0.772591931467384,55.7451294709179,-2.47780062126731));
#10643=CARTESIAN_POINT('Origin',(0.780904059217543,56.2445672509427,-2.49999999999999));
#10644=CARTESIAN_POINT('',(0.780904059217487,56.2445672509427,-2.));
#10645=CARTESIAN_POINT('Origin',(0.780904059217543,56.2445672509427,-2.49999999999999));
#10646=CARTESIAN_POINT('Origin',(0.780904059217543,56.2445672509427,-2.49999999999999));
#10647=CARTESIAN_POINT('Origin',(0.7809040592178,56.2445672509427,2.5));
#10648=CARTESIAN_POINT('Origin',(0.7809040592178,56.2445672509427,2.5));
#10649=CARTESIAN_POINT('Ctrl Pts',(0.179907800164864,56.095149243924,-2.48301423187597));
#10650=CARTESIAN_POINT('Ctrl Pts',(0.273542643066175,56.0170448409569,-2.4829907879535));
#10651=CARTESIAN_POINT('Ctrl Pts',(0.367177330124766,55.9389402576095,-2.48296724699913));
#10652=CARTESIAN_POINT('Ctrl Pts',(0.460811859385246,55.8608354916479,-2.48294360779847));
#10653=CARTESIAN_POINT('Ctrl Pts',(0.182694641762887,56.0984901824412,-2.3550199649901));
#10654=CARTESIAN_POINT('Ctrl Pts',(0.276333332478466,56.0203903852817,-2.35500062661495));
#10655=CARTESIAN_POINT('Ctrl Pts',(0.369971635899436,55.9422901242086,-2.35498122632127));
#10656=CARTESIAN_POINT('Ctrl Pts',(0.46361004433911,55.8641900014914,-2.35496172772305));
#10657=CARTESIAN_POINT('Ctrl Pts',(0.254541365578152,56.1846219120289,-2.1035560356539));
#10658=CARTESIAN_POINT('Ctrl Pts',(0.348183189883077,56.1065256357555,-2.10354935262451));
#10659=CARTESIAN_POINT('Ctrl Pts',(0.441824994766326,56.0284293435915,-2.10354276030279));
#10660=CARTESIAN_POINT('Ctrl Pts',(0.535466562098709,55.9503327690789,-2.1035360223157));
#10661=CARTESIAN_POINT('Ctrl Pts',(0.417965393799912,56.380538906701,-2.));
#10662=CARTESIAN_POINT('Ctrl Pts',(0.51160263229286,56.3024366043021,-2.00000011921147));
#10663=CARTESIAN_POINT('Ctrl Pts',(0.605239657990597,56.224334047085,-1.99999987982882));
#10664=CARTESIAN_POINT('Ctrl Pts',(0.698876602273422,56.1462313952734,-2.00000000000001));
#10665=CARTESIAN_POINT('Ctrl Pts',(0.499999999997104,56.4788841358583,-2.));
#10666=CARTESIAN_POINT('Ctrl Pts',(0.593634842898415,56.4007786951616,-2.));
#10667=CARTESIAN_POINT('Ctrl Pts',(0.687269529957005,56.3226730676371,-2.00000000000001));
#10668=CARTESIAN_POINT('Ctrl Pts',(0.780904059217486,56.2445672509429,-2.00000000000001));
#10669=CARTESIAN_POINT('Ctrl Pts',(0.179907800164864,56.095149243924,-2.48301423187597));
#10670=CARTESIAN_POINT('Ctrl Pts',(0.273542643066175,56.0170448409569,-2.4829907879535));
#10671=CARTESIAN_POINT('Ctrl Pts',(0.367177330124766,55.9389402576095,-2.48296724699913));
#10672=CARTESIAN_POINT('Ctrl Pts',(0.460811859385246,55.8608354916479,-2.48294360779847));
#10673=CARTESIAN_POINT('Ctrl Pts',(0.780904059217486,56.2445672509429,-2.00000000000001));
#10674=CARTESIAN_POINT('Ctrl Pts',(0.687269529957005,56.3226730676371,-2.00000000000001));
#10675=CARTESIAN_POINT('Ctrl Pts',(0.593634842898415,56.4007786951616,-2.));
#10676=CARTESIAN_POINT('Ctrl Pts',(0.499999999997104,56.4788841358583,-2.));
#10677=CARTESIAN_POINT('Ctrl Pts',(3.30000000000011,55.3431808226541,-2.));
#10678=CARTESIAN_POINT('Ctrl Pts',(2.61488947773062,55.9545258328107,-2.));
#10679=CARTESIAN_POINT('Ctrl Pts',(1.68855421348719,56.2382465200534,-2.));
#10680=CARTESIAN_POINT('Ctrl Pts',(0.780904059217557,56.2445672509427,-2.));
#10681=CARTESIAN_POINT('Ctrl Pts',(3.12847993397321,55.1464989588649,-1.99359023604657));
#10682=CARTESIAN_POINT('Ctrl Pts',(2.49435860108456,55.7131228937494,-1.99369822098603));
#10683=CARTESIAN_POINT('Ctrl Pts',(1.6423051555987,55.9779696257069,-1.99374127621725));
#10684=CARTESIAN_POINT('Ctrl Pts',(0.776592785321963,55.985522499928,-1.99373831640894));
#10685=CARTESIAN_POINT('Ctrl Pts',(2.97318977758963,54.9684279139248,-2.22195490734826));
#10686=CARTESIAN_POINT('Ctrl Pts',(2.38493152738063,55.4942042697613,-2.219584961608));
#10687=CARTESIAN_POINT('Ctrl Pts',(1.60032112558294,55.7416794204833,-2.2186313537272));
#10688=CARTESIAN_POINT('Ctrl Pts',(0.772679250843375,55.750376093287,-2.21869746782962));
#10689=CARTESIAN_POINT('Ctrl Pts',(2.97156409628604,54.9665637470309,-2.4829871959822));
#10690=CARTESIAN_POINT('Ctrl Pts',(2.3824255311525,55.4902988970164,-2.47922636145333));
#10691=CARTESIAN_POINT('Ctrl Pts',(1.59937395537643,55.7362908562734,-2.47769302204319));
#10692=CARTESIAN_POINT('Ctrl Pts',(0.772591931467199,55.7451294709179,-2.47780062126726));
#10693=CARTESIAN_POINT('',(2.971564096286,54.9665637470309,-2.48298719598216));
#10694=CARTESIAN_POINT('Ctrl Pts',(0.772591931467199,55.7451294709179,-2.47780062126726));
#10695=CARTESIAN_POINT('Ctrl Pts',(1.59937395537643,55.7362908562734,-2.47769302204319));
#10696=CARTESIAN_POINT('Ctrl Pts',(2.3824255311525,55.4902988970164,-2.47922636145333));
#10697=CARTESIAN_POINT('Ctrl Pts',(2.97156409628604,54.9665637470309,-2.4829871959822));
#10698=CARTESIAN_POINT('',(2.8,55.359994587709,-2.09491355855718));
#10699=CARTESIAN_POINT('Ctrl Pts',(2.971564096286,54.9665637470309,-2.4829871959822));
#10700=CARTESIAN_POINT('Ctrl Pts',(2.97105810082493,54.9670227222473,-2.48226197818885));
#10701=CARTESIAN_POINT('Ctrl Pts',(2.97055313800993,54.9674828549434,-2.48153699974797));
#10702=CARTESIAN_POINT('Ctrl Pts',(2.97004920764725,54.9679441397298,-2.48081226422373));
#10703=CARTESIAN_POINT('Ctrl Pts',(2.95167041222309,54.9847676124758,-2.45438050514927));
#10704=CARTESIAN_POINT('Ctrl Pts',(2.9345112351927,55.003258903751,-2.42807817015696));
#10705=CARTESIAN_POINT('Ctrl Pts',(2.91866949298605,55.0232080767984,-2.4020995131002));
#10706=CARTESIAN_POINT('Ctrl Pts',(2.90322420614785,55.0426580019318,-2.37677099779685));
#10707=CARTESIAN_POINT('Ctrl Pts',(2.8890308989744,55.0634947711076,-2.35174970589681));
#10708=CARTESIAN_POINT('Ctrl Pts',(2.87621470782766,55.085540523235,-2.32724566770674));
#10709=CARTESIAN_POINT('Ctrl Pts',(2.86402565276861,55.1065075081544,-2.30394068830622));
#10710=CARTESIAN_POINT('Ctrl Pts',(2.85308218625054,55.1285688920359,-2.28110332092758));
#10711=CARTESIAN_POINT('Ctrl Pts',(2.8435260528693,55.1515737238906,-2.25894659880361));
#10712=CARTESIAN_POINT('Ctrl Pts',(2.84019421835236,55.1595945718394,-2.25122145217687));
#10713=CARTESIAN_POINT('Ctrl Pts',(2.83703135085799,55.1677300706399,-2.24357936415525));
#10714=CARTESIAN_POINT('Ctrl Pts',(2.83404451182727,55.1759736024566,-2.23603044811829));
#10715=CARTESIAN_POINT('Ctrl Pts',(2.82677792422061,55.1960290341415,-2.21766492551939));
#10716=CARTESIAN_POINT('Ctrl Pts',(2.82047457316189,55.2169382222468,-2.19965231451423));
#10717=CARTESIAN_POINT('Ctrl Pts',(2.8153526628751,55.2386030649626,-2.18220983334552));
#10718=CARTESIAN_POINT('Ctrl Pts',(2.81055920641232,55.2588786017284,-2.16588588985499));
#10719=CARTESIAN_POINT('Ctrl Pts',(2.80680052944647,55.2798164625832,-2.15006131614833));
#10720=CARTESIAN_POINT('Ctrl Pts',(2.8042702594812,55.3013208330089,-2.13495270927354));
#10721=CARTESIAN_POINT('Ctrl Pts',(2.80195466870913,55.3210006784011,-2.1211259828221));
#10722=CARTESIAN_POINT('Ctrl Pts',(2.80066799680603,55.3411552064162,-2.10789905750761));
#10723=CARTESIAN_POINT('Ctrl Pts',(2.8005704592906,55.3616930895013,-2.09546976536745));
#10724=CARTESIAN_POINT('',(2.79999999653565,55.7079964402821,-2.));
#10725=CARTESIAN_POINT('Ctrl Pts',(2.79999999999999,55.359994587709,-2.09491355855717));
#10726=CARTESIAN_POINT('Ctrl Pts',(2.79999999999999,55.3882860920536,-2.07799898836919));
#10727=CARTESIAN_POINT('Ctrl Pts',(2.80000000000001,55.4179318200166,-2.0632732682766));
#10728=CARTESIAN_POINT('Ctrl Pts',(2.80000000000001,55.530483252799,-2.01733304327692));
#10729=CARTESIAN_POINT('Ctrl Pts',(2.79999999999996,55.6192843749741,-2.));
#10730=CARTESIAN_POINT('Ctrl Pts',(2.79999999999996,55.7079964361128,-2.));
#10731=CARTESIAN_POINT('Ctrl Pts',(2.80000021990589,55.7079968150647,-1.99998051174467));
#10732=CARTESIAN_POINT('Ctrl Pts',(2.1959878240584,56.0680119999874,-1.99998070337318));
#10733=CARTESIAN_POINT('Ctrl Pts',(1.48287989181725,56.2388471215568,-1.99998078197634));
#10734=CARTESIAN_POINT('Ctrl Pts',(0.780890281868511,56.2437394329846,-1.9999807748488));
#10735=CARTESIAN_POINT('Ctrl Pts',(0.6,55.8,0.));
#10736=CARTESIAN_POINT('Ctrl Pts',(0.6,55.8,55.8));
#10737=CARTESIAN_POINT('Ctrl Pts',(0.600000000000001,0.,55.8));
#10738=CARTESIAN_POINT('Ctrl Pts',(0.600000000000001,-55.8,55.8));
#10739=CARTESIAN_POINT('Ctrl Pts',(0.600000000000001,-55.8,0.));
#10740=CARTESIAN_POINT('Ctrl Pts',(0.600000000000001,-55.8,-55.8));
#10741=CARTESIAN_POINT('Ctrl Pts',(0.600000000000001,0.,-55.8));
#10742=CARTESIAN_POINT('Ctrl Pts',(0.6,55.8,-55.8));
#10743=CARTESIAN_POINT('Ctrl Pts',(0.6,55.8,0.));
#10744=CARTESIAN_POINT('Ctrl Pts',(0.701236460530903,55.8018466247247,0.));
#10745=CARTESIAN_POINT('Ctrl Pts',(0.701236460530903,55.8018466247247,55.8018466247247));
#10746=CARTESIAN_POINT('Ctrl Pts',(0.701236460530903,0.,55.8018466247247));
#10747=CARTESIAN_POINT('Ctrl Pts',(0.701236460530903,-55.8018466247247,
55.8018466247247));
#10748=CARTESIAN_POINT('Ctrl Pts',(0.701236460530903,-55.8018466247247,
0.));
#10749=CARTESIAN_POINT('Ctrl Pts',(0.701236460530903,-55.8018466247247,
-55.8018466247247));
#10750=CARTESIAN_POINT('Ctrl Pts',(0.701236460530903,0.,-55.8018466247247));
#10751=CARTESIAN_POINT('Ctrl Pts',(0.701236460530903,55.8018466247247,-55.8018466247247));
#10752=CARTESIAN_POINT('Ctrl Pts',(0.701236460530903,55.8018466247247,0.));
#10753=CARTESIAN_POINT('Ctrl Pts',(0.900815345510183,55.8004649202247,0.));
#10754=CARTESIAN_POINT('Ctrl Pts',(0.900815345510183,55.8004649202247,55.8004649202247));
#10755=CARTESIAN_POINT('Ctrl Pts',(0.900815345510182,0.,55.8004649202247));
#10756=CARTESIAN_POINT('Ctrl Pts',(0.900815345510181,-55.8004649202247,
55.8004649202247));
#10757=CARTESIAN_POINT('Ctrl Pts',(0.900815345510181,-55.8004649202247,
0.));
#10758=CARTESIAN_POINT('Ctrl Pts',(0.900815345510181,-55.8004649202247,
-55.8004649202247));
#10759=CARTESIAN_POINT('Ctrl Pts',(0.900815345510182,0.,-55.8004649202247));
#10760=CARTESIAN_POINT('Ctrl Pts',(0.900815345510183,55.8004649202247,-55.8004649202247));
#10761=CARTESIAN_POINT('Ctrl Pts',(0.900815345510183,55.8004649202247,0.));
#10762=CARTESIAN_POINT('Ctrl Pts',(1.1915014799956,55.7831674035309,0.));
#10763=CARTESIAN_POINT('Ctrl Pts',(1.1915014799956,55.7831674035309,55.7831674035309));
#10764=CARTESIAN_POINT('Ctrl Pts',(1.1915014799956,0.,55.7831674035309));
#10765=CARTESIAN_POINT('Ctrl Pts',(1.1915014799956,-55.7831674035309,55.7831674035309));
#10766=CARTESIAN_POINT('Ctrl Pts',(1.1915014799956,-55.7831674035309,0.));
#10767=CARTESIAN_POINT('Ctrl Pts',(1.1915014799956,-55.7831674035309,-55.7831674035309));
#10768=CARTESIAN_POINT('Ctrl Pts',(1.1915014799956,0.,-55.7831674035309));
#10769=CARTESIAN_POINT('Ctrl Pts',(1.1915014799956,55.7831674035309,-55.7831674035309));
#10770=CARTESIAN_POINT('Ctrl Pts',(1.1915014799956,55.7831674035309,0.));
#10771=CARTESIAN_POINT('Ctrl Pts',(1.56159311954184,55.7294336445653,0.));
#10772=CARTESIAN_POINT('Ctrl Pts',(1.56159311954184,55.7294336445653,55.7294336445653));
#10773=CARTESIAN_POINT('Ctrl Pts',(1.56159311954184,0.,55.7294336445653));
#10774=CARTESIAN_POINT('Ctrl Pts',(1.56159311954184,-55.7294336445653,55.7294336445653));
#10775=CARTESIAN_POINT('Ctrl Pts',(1.56159311954184,-55.7294336445653,0.));
#10776=CARTESIAN_POINT('Ctrl Pts',(1.56159311954184,-55.7294336445653,-55.7294336445653));
#10777=CARTESIAN_POINT('Ctrl Pts',(1.56159311954184,0.,-55.7294336445653));
#10778=CARTESIAN_POINT('Ctrl Pts',(1.56159311954184,55.7294336445653,-55.7294336445653));
#10779=CARTESIAN_POINT('Ctrl Pts',(1.56159311954184,55.7294336445653,0.));
#10780=CARTESIAN_POINT('Ctrl Pts',(1.99433075254501,55.6097757263875,0.));
#10781=CARTESIAN_POINT('Ctrl Pts',(1.99433075254501,55.6097757263875,55.6097757263875));
#10782=CARTESIAN_POINT('Ctrl Pts',(1.99433075254501,0.,55.6097757263875));
#10783=CARTESIAN_POINT('Ctrl Pts',(1.99433075254501,-55.6097757263875,55.6097757263875));
#10784=CARTESIAN_POINT('Ctrl Pts',(1.99433075254501,-55.6097757263875,0.));
#10785=CARTESIAN_POINT('Ctrl Pts',(1.99433075254501,-55.6097757263875,-55.6097757263875));
#10786=CARTESIAN_POINT('Ctrl Pts',(1.99433075254501,0.,-55.6097757263875));
#10787=CARTESIAN_POINT('Ctrl Pts',(1.99433075254501,55.6097757263875,-55.6097757263875));
#10788=CARTESIAN_POINT('Ctrl Pts',(1.99433075254501,55.6097757263875,0.));
#10789=CARTESIAN_POINT('Ctrl Pts',(2.39636115062391,55.4358658864373,0.));
#10790=CARTESIAN_POINT('Ctrl Pts',(2.39636115062391,55.4358658864373,55.4358658864373));
#10791=CARTESIAN_POINT('Ctrl Pts',(2.39636115062391,0.,55.4358658864373));
#10792=CARTESIAN_POINT('Ctrl Pts',(2.39636115062391,-55.4358658864373,55.4358658864373));
#10793=CARTESIAN_POINT('Ctrl Pts',(2.39636115062391,-55.4358658864373,0.));
#10794=CARTESIAN_POINT('Ctrl Pts',(2.39636115062391,-55.4358658864373,-55.4358658864373));
#10795=CARTESIAN_POINT('Ctrl Pts',(2.39636115062391,0.,-55.4358658864373));
#10796=CARTESIAN_POINT('Ctrl Pts',(2.39636115062391,55.4358658864373,-55.4358658864373));
#10797=CARTESIAN_POINT('Ctrl Pts',(2.39636115062391,55.4358658864373,0.));
#10798=CARTESIAN_POINT('Ctrl Pts',(2.7670687050864,55.2060224359905,0.));
#10799=CARTESIAN_POINT('Ctrl Pts',(2.7670687050864,55.2060224359905,55.2060224359905));
#10800=CARTESIAN_POINT('Ctrl Pts',(2.7670687050864,0.,55.2060224359905));
#10801=CARTESIAN_POINT('Ctrl Pts',(2.7670687050864,-55.2060224359905,55.2060224359905));
#10802=CARTESIAN_POINT('Ctrl Pts',(2.7670687050864,-55.2060224359905,0.));
#10803=CARTESIAN_POINT('Ctrl Pts',(2.7670687050864,-55.2060224359905,-55.2060224359905));
#10804=CARTESIAN_POINT('Ctrl Pts',(2.7670687050864,0.,-55.2060224359905));
#10805=CARTESIAN_POINT('Ctrl Pts',(2.7670687050864,55.2060224359905,-55.2060224359905));
#10806=CARTESIAN_POINT('Ctrl Pts',(2.7670687050864,55.2060224359905,0.));
#10807=CARTESIAN_POINT('Ctrl Pts',(3.10660035178773,54.9194536393824,0.));
#10808=CARTESIAN_POINT('Ctrl Pts',(3.10660035178773,54.9194536393824,54.9194536393824));
#10809=CARTESIAN_POINT('Ctrl Pts',(3.10660035178772,0.,54.9194536393824));
#10810=CARTESIAN_POINT('Ctrl Pts',(3.10660035178772,-54.9194536393824,54.9194536393824));
#10811=CARTESIAN_POINT('Ctrl Pts',(3.10660035178772,-54.9194536393824,0.));
#10812=CARTESIAN_POINT('Ctrl Pts',(3.10660035178772,-54.9194536393824,-54.9194536393824));
#10813=CARTESIAN_POINT('Ctrl Pts',(3.10660035178772,0.,-54.9194536393824));
#10814=CARTESIAN_POINT('Ctrl Pts',(3.10660035178773,54.9194536393824,-54.9194536393824));
#10815=CARTESIAN_POINT('Ctrl Pts',(3.10660035178773,54.9194536393824,0.));
#10816=CARTESIAN_POINT('Ctrl Pts',(3.41599349838964,54.5765115223889,0.));
#10817=CARTESIAN_POINT('Ctrl Pts',(3.41599349838964,54.5765115223889,54.5765115223889));
#10818=CARTESIAN_POINT('Ctrl Pts',(3.41599349838964,0.,54.5765115223889));
#10819=CARTESIAN_POINT('Ctrl Pts',(3.41599349838964,-54.5765115223889,54.5765115223889));
#10820=CARTESIAN_POINT('Ctrl Pts',(3.41599349838964,-54.5765115223889,0.));
#10821=CARTESIAN_POINT('Ctrl Pts',(3.41599349838964,-54.5765115223889,-54.5765115223889));
#10822=CARTESIAN_POINT('Ctrl Pts',(3.41599349838964,0.,-54.5765115223889));
#10823=CARTESIAN_POINT('Ctrl Pts',(3.41599349838964,54.5765115223889,-54.5765115223889));
#10824=CARTESIAN_POINT('Ctrl Pts',(3.41599349838964,54.5765115223889,0.));
#10825=CARTESIAN_POINT('Ctrl Pts',(3.69673657250524,54.1781787924237,0.));
#10826=CARTESIAN_POINT('Ctrl Pts',(3.69673657250524,54.1781787924237,54.1781787924237));
#10827=CARTESIAN_POINT('Ctrl Pts',(3.69673657250524,0.,54.1781787924237));
#10828=CARTESIAN_POINT('Ctrl Pts',(3.69673657250524,-54.1781787924237,54.1781787924237));
#10829=CARTESIAN_POINT('Ctrl Pts',(3.69673657250524,-54.1781787924237,0.));
#10830=CARTESIAN_POINT('Ctrl Pts',(3.69673657250524,-54.1781787924237,-54.1781787924237));
#10831=CARTESIAN_POINT('Ctrl Pts',(3.69673657250524,0.,-54.1781787924237));
#10832=CARTESIAN_POINT('Ctrl Pts',(3.69673657250524,54.1781787924237,-54.1781787924237));
#10833=CARTESIAN_POINT('Ctrl Pts',(3.69673657250524,54.1781787924237,0.));
#10834=CARTESIAN_POINT('Ctrl Pts',(3.95058412182039,53.7259602136685,0.));
#10835=CARTESIAN_POINT('Ctrl Pts',(3.95058412182039,53.7259602136685,53.7259602136685));
#10836=CARTESIAN_POINT('Ctrl Pts',(3.95058412182039,0.,53.7259602136685));
#10837=CARTESIAN_POINT('Ctrl Pts',(3.95058412182039,-53.7259602136685,53.7259602136685));
#10838=CARTESIAN_POINT('Ctrl Pts',(3.95058412182039,-53.7259602136685,0.));
#10839=CARTESIAN_POINT('Ctrl Pts',(3.95058412182039,-53.7259602136685,-53.7259602136685));
#10840=CARTESIAN_POINT('Ctrl Pts',(3.95058412182039,0.,-53.7259602136685));
#10841=CARTESIAN_POINT('Ctrl Pts',(3.95058412182039,53.7259602136685,-53.7259602136685));
#10842=CARTESIAN_POINT('Ctrl Pts',(3.95058412182039,53.7259602136685,0.));
#10843=CARTESIAN_POINT('Ctrl Pts',(4.17937157605894,53.2217823983375,0.));
#10844=CARTESIAN_POINT('Ctrl Pts',(4.17937157605894,53.2217823983375,53.2217823983375));
#10845=CARTESIAN_POINT('Ctrl Pts',(4.17937157605894,0.,53.2217823983375));
#10846=CARTESIAN_POINT('Ctrl Pts',(4.17937157605894,-53.2217823983375,53.2217823983375));
#10847=CARTESIAN_POINT('Ctrl Pts',(4.17937157605894,-53.2217823983375,0.));
#10848=CARTESIAN_POINT('Ctrl Pts',(4.17937157605894,-53.2217823983375,-53.2217823983375));
#10849=CARTESIAN_POINT('Ctrl Pts',(4.17937157605894,0.,-53.2217823983375));
#10850=CARTESIAN_POINT('Ctrl Pts',(4.17937157605894,53.2217823983375,-53.2217823983375));
#10851=CARTESIAN_POINT('Ctrl Pts',(4.17937157605894,53.2217823983375,0.));
#10852=CARTESIAN_POINT('Ctrl Pts',(4.38495097171173,52.6681920799401,0.));
#10853=CARTESIAN_POINT('Ctrl Pts',(4.38495097171173,52.6681920799401,52.6681920799401));
#10854=CARTESIAN_POINT('Ctrl Pts',(4.38495097171173,0.,52.6681920799401));
#10855=CARTESIAN_POINT('Ctrl Pts',(4.38495097171173,-52.6681920799401,52.6681920799401));
#10856=CARTESIAN_POINT('Ctrl Pts',(4.38495097171173,-52.6681920799401,0.));
#10857=CARTESIAN_POINT('Ctrl Pts',(4.38495097171173,-52.6681920799401,-52.6681920799401));
#10858=CARTESIAN_POINT('Ctrl Pts',(4.38495097171173,0.,-52.6681920799401));
#10859=CARTESIAN_POINT('Ctrl Pts',(4.38495097171173,52.6681920799401,-52.6681920799401));
#10860=CARTESIAN_POINT('Ctrl Pts',(4.38495097171173,52.6681920799401,0.));
#10861=CARTESIAN_POINT('Ctrl Pts',(4.56903002475152,52.0679652261342,0.));
#10862=CARTESIAN_POINT('Ctrl Pts',(4.56903002475152,52.0679652261342,52.0679652261342));
#10863=CARTESIAN_POINT('Ctrl Pts',(4.56903002475152,0.,52.0679652261342));
#10864=CARTESIAN_POINT('Ctrl Pts',(4.56903002475152,-52.0679652261342,52.0679652261342));
#10865=CARTESIAN_POINT('Ctrl Pts',(4.56903002475152,-52.0679652261342,0.));
#10866=CARTESIAN_POINT('Ctrl Pts',(4.56903002475152,-52.0679652261342,-52.0679652261342));
#10867=CARTESIAN_POINT('Ctrl Pts',(4.56903002475152,0.,-52.0679652261342));
#10868=CARTESIAN_POINT('Ctrl Pts',(4.56903002475152,52.0679652261342,-52.0679652261342));
#10869=CARTESIAN_POINT('Ctrl Pts',(4.56903002475152,52.0679652261342,0.));
#10870=CARTESIAN_POINT('Ctrl Pts',(4.73302863242595,51.423645039376,0.));
#10871=CARTESIAN_POINT('Ctrl Pts',(4.73302863242595,51.423645039376,51.423645039376));
#10872=CARTESIAN_POINT('Ctrl Pts',(4.73302863242595,0.,51.423645039376));
#10873=CARTESIAN_POINT('Ctrl Pts',(4.73302863242595,-51.423645039376,51.423645039376));
#10874=CARTESIAN_POINT('Ctrl Pts',(4.73302863242595,-51.423645039376,0.));
#10875=CARTESIAN_POINT('Ctrl Pts',(4.73302863242595,-51.423645039376,-51.423645039376));
#10876=CARTESIAN_POINT('Ctrl Pts',(4.73302863242595,0.,-51.423645039376));
#10877=CARTESIAN_POINT('Ctrl Pts',(4.73302863242595,51.423645039376,-51.423645039376));
#10878=CARTESIAN_POINT('Ctrl Pts',(4.73302863242595,51.423645039376,0.));
#10879=CARTESIAN_POINT('Ctrl Pts',(4.84900124161322,50.8745342238058,0.));
#10880=CARTESIAN_POINT('Ctrl Pts',(4.84900124161322,50.8745342238058,50.8745342238058));
#10881=CARTESIAN_POINT('Ctrl Pts',(4.84900124161322,0.,50.8745342238058));
#10882=CARTESIAN_POINT('Ctrl Pts',(4.84900124161322,-50.8745342238058,50.8745342238058));
#10883=CARTESIAN_POINT('Ctrl Pts',(4.84900124161322,-50.8745342238058,0.));
#10884=CARTESIAN_POINT('Ctrl Pts',(4.84900124161322,-50.8745342238058,-50.8745342238058));
#10885=CARTESIAN_POINT('Ctrl Pts',(4.84900124161322,0.,-50.8745342238058));
#10886=CARTESIAN_POINT('Ctrl Pts',(4.84900124161322,50.8745342238058,-50.8745342238058));
#10887=CARTESIAN_POINT('Ctrl Pts',(4.84900124161322,50.8745342238058,0.));
#10888=CARTESIAN_POINT('Ctrl Pts',(4.92769824210582,50.4443513809858,0.));
#10889=CARTESIAN_POINT('Ctrl Pts',(4.92769824210582,50.4443513809858,50.4443513809858));
#10890=CARTESIAN_POINT('Ctrl Pts',(4.92769824210582,0.,50.4443513809858));
#10891=CARTESIAN_POINT('Ctrl Pts',(4.92769824210582,-50.4443513809858,50.4443513809858));
#10892=CARTESIAN_POINT('Ctrl Pts',(4.92769824210582,-50.4443513809858,0.));
#10893=CARTESIAN_POINT('Ctrl Pts',(4.92769824210582,-50.4443513809858,-50.4443513809858));
#10894=CARTESIAN_POINT('Ctrl Pts',(4.92769824210582,0.,-50.4443513809858));
#10895=CARTESIAN_POINT('Ctrl Pts',(4.92769824210582,50.4443513809858,-50.4443513809858));
#10896=CARTESIAN_POINT('Ctrl Pts',(4.92769824210582,50.4443513809858,0.));
#10897=CARTESIAN_POINT('Ctrl Pts',(4.97650848841056,50.1494665212081,0.));
#10898=CARTESIAN_POINT('Ctrl Pts',(4.97650848841056,50.1494665212081,50.1494665212081));
#10899=CARTESIAN_POINT('Ctrl Pts',(4.97650848841056,0.,50.1494665212081));
#10900=CARTESIAN_POINT('Ctrl Pts',(4.97650848841056,-50.1494665212081,50.1494665212081));
#10901=CARTESIAN_POINT('Ctrl Pts',(4.97650848841056,-50.1494665212081,0.));
#10902=CARTESIAN_POINT('Ctrl Pts',(4.97650848841056,-50.1494665212081,-50.1494665212081));
#10903=CARTESIAN_POINT('Ctrl Pts',(4.97650848841056,0.,-50.1494665212081));
#10904=CARTESIAN_POINT('Ctrl Pts',(4.97650848841056,50.1494665212081,-50.1494665212081));
#10905=CARTESIAN_POINT('Ctrl Pts',(4.97650848841056,50.1494665212081,0.));
#10906=CARTESIAN_POINT('Ctrl Pts',(5.,50.,0.));
#10907=CARTESIAN_POINT('Ctrl Pts',(5.,50.,50.));
#10908=CARTESIAN_POINT('Ctrl Pts',(5.,0.,50.));
#10909=CARTESIAN_POINT('Ctrl Pts',(5.,-50.,50.));
#10910=CARTESIAN_POINT('Ctrl Pts',(5.,-50.,0.));
#10911=CARTESIAN_POINT('Ctrl Pts',(5.,-50.,-50.));
#10912=CARTESIAN_POINT('Ctrl Pts',(5.,0.,-50.));
#10913=CARTESIAN_POINT('Ctrl Pts',(5.,50.,-50.));
#10914=CARTESIAN_POINT('Ctrl Pts',(5.,50.,0.));
#10915=CARTESIAN_POINT('',(2.97156409628618,54.9665637470307,2.48298719598219));
#10916=CARTESIAN_POINT('Ctrl Pts',(2.97156409628618,54.9665637470307,2.48298719598219));
#10917=CARTESIAN_POINT('Ctrl Pts',(2.38240222522867,55.4903197198984,2.47922620961122));
#10918=CARTESIAN_POINT('Ctrl Pts',(1.59934858958684,55.7362874995129,2.47769305658212));
#10919=CARTESIAN_POINT('Ctrl Pts',(0.772591931467188,55.7451294709179,2.47780062126727));
#10920=CARTESIAN_POINT('',(2.97156409628601,55.0226167641255,6.66133814775094E-15));
#10921=CARTESIAN_POINT('Ctrl Pts',(2.971564096286,55.0226075943045,1.82631687550838E-14));
#10922=CARTESIAN_POINT('Ctrl Pts',(2.971564096286,55.0226075940038,0.827947557198553));
#10923=CARTESIAN_POINT('Ctrl Pts',(2.97156409628599,55.0039260136328,1.65588852538752));
#10924=CARTESIAN_POINT('Ctrl Pts',(2.97156409628599,54.9665637470306,2.48298719598933));
#10925=CARTESIAN_POINT('',(4.99841192763649,50.010089934565,-1.0547118733939E-14));
#10926=CARTESIAN_POINT('Ctrl Pts',(4.99841192763651,50.0100899345649,0.));
#10927=CARTESIAN_POINT('Ctrl Pts',(4.97518900611397,50.157429856102,0.));
#10928=CARTESIAN_POINT('Ctrl Pts',(4.92663484069112,50.450160402527,0.));
#10929=CARTESIAN_POINT('Ctrl Pts',(4.84821789314001,50.8782420415372,0.));
#10930=CARTESIAN_POINT('Ctrl Pts',(4.73258563268563,51.4253855033925,0.));
#10931=CARTESIAN_POINT('Ctrl Pts',(4.56903002475152,52.0679652261342,0.));
#10932=CARTESIAN_POINT('Ctrl Pts',(4.38495097171173,52.6681920799401,0.));
#10933=CARTESIAN_POINT('Ctrl Pts',(4.17937157605894,53.2217823983375,0.));
#10934=CARTESIAN_POINT('Ctrl Pts',(3.95058412182039,53.7259602136685,0.));
#10935=CARTESIAN_POINT('Ctrl Pts',(3.69673657250524,54.1781787924237,0.));
#10936=CARTESIAN_POINT('Ctrl Pts',(3.45047359613994,54.527589384204,0.));
#10937=CARTESIAN_POINT('Ctrl Pts',(3.24393642390649,54.765582391618,0.));
#10938=CARTESIAN_POINT('Ctrl Pts',(3.08990662218085,54.9172980064984,0.));
#10939=CARTESIAN_POINT('Ctrl Pts',(2.99751746911325,55.0000067011129,0.));
#10940=CARTESIAN_POINT('Ctrl Pts',(2.97156409628601,55.0226167641255,0.));
#10941=CARTESIAN_POINT('Ctrl Pts',(4.99841192763649,50.0100899345651,-2.44355213456396E-14));
#10942=CARTESIAN_POINT('Ctrl Pts',(4.99841192763649,50.010089934565,-7.48115762363152));
#10943=CARTESIAN_POINT('Ctrl Pts',(4.9984119276365,46.6017252207067,-22.4413792780267));
#10944=CARTESIAN_POINT('Ctrl Pts',(4.99841192763649,33.8387987663498,-38.4316981785149));
#10945=CARTESIAN_POINT('Ctrl Pts',(4.9984119276365,18.5446192921948,-47.2509187816055));
#10946=CARTESIAN_POINT('Ctrl Pts',(4.99841192763649,6.25354094871083,-50.0596743547279));
#10947=CARTESIAN_POINT('Ctrl Pts',(4.99841192763649,-3.75050037564627,-50.055717263026));
#10948=CARTESIAN_POINT('Ctrl Pts',(4.99841192763649,-13.6423328766374,-48.5678652060244));
#10949=CARTESIAN_POINT('Ctrl Pts',(4.9984119276365,-25.3805953459256,-43.9618581545187));
#10950=CARTESIAN_POINT('Ctrl Pts',(4.99841192763649,-37.210931604044,-34.5275648165732));
#10951=CARTESIAN_POINT('Ctrl Pts',(4.99841192763649,-45.7357692537155,-22.0258961118735));
#10952=CARTESIAN_POINT('Ctrl Pts',(4.9984119276365,-50.1946948077045,-7.566025938944));
#10953=CARTESIAN_POINT('Ctrl Pts',(4.9984119276365,-50.1960569239472,7.56522373629383));
#10954=CARTESIAN_POINT('Ctrl Pts',(4.99841192763649,-45.7352070158957,22.0246092149029));
#10955=CARTESIAN_POINT('Ctrl Pts',(4.99841192763649,-37.2116055718427,34.5267335901821));
#10956=CARTESIAN_POINT('Ctrl Pts',(4.99841192763649,-25.3814385247641,43.9614029395442));
#10957=CARTESIAN_POINT('Ctrl Pts',(4.99841192763649,-11.2963143151676,49.4899240087747));
#10958=CARTESIAN_POINT('Ctrl Pts',(4.99841192763649,3.7937298863526,50.6205829747067));
#10959=CARTESIAN_POINT('Ctrl Pts',(4.99841192763649,18.5440439702159,47.2521255691362));
#10960=CARTESIAN_POINT('Ctrl Pts',(4.99841192763649,33.8380966958625,38.4319339724568));
#10961=CARTESIAN_POINT('Ctrl Pts',(4.9984119276365,46.6012579438089,22.4429169923092));
#10962=CARTESIAN_POINT('Ctrl Pts',(4.99841192763649,50.010089934565,7.48115762363149));
#10963=CARTESIAN_POINT('Ctrl Pts',(4.99841192763649,50.010089934565,-2.22455486416984E-15));
#10964=CARTESIAN_POINT('Ctrl Pts',(2.971564096286,54.9665637470309,-2.48298719598223));
#10965=CARTESIAN_POINT('Ctrl Pts',(2.971564096286,55.0039266101128,-1.65587532094447));
#10966=CARTESIAN_POINT('Ctrl Pts',(2.971564096286,55.0226075946053,-0.827934366072422));
#10967=CARTESIAN_POINT('Ctrl Pts',(2.971564096286,55.0226075943045,1.82631687550838E-14));
#10968=CARTESIAN_POINT('Ctrl Pts',(0.780904059217545,56.2445672509427,2.));
#10969=CARTESIAN_POINT('Ctrl Pts',(1.68852632773542,56.2382423732899,2.));
#10970=CARTESIAN_POINT('Ctrl Pts',(2.61486131739033,55.9545502327436,2.));
#10971=CARTESIAN_POINT('Ctrl Pts',(3.30000000000027,55.3431808226539,2.));
#10972=CARTESIAN_POINT('Ctrl Pts',(0.776592785321951,55.9855224999279,1.99373831640894));
#10973=CARTESIAN_POINT('Ctrl Pts',(1.64227856307928,55.977965882459,1.99374127522468));
#10974=CARTESIAN_POINT('Ctrl Pts',(2.49433299618752,55.7131454773729,1.99369822532176));
#10975=CARTESIAN_POINT('Ctrl Pts',(3.12847993397336,55.1464989588648,1.99359023604657));
#10976=CARTESIAN_POINT('Ctrl Pts',(0.772679250843364,55.750376093287,2.21869746782962));
#10977=CARTESIAN_POINT('Ctrl Pts',(1.60029571178559,55.741676045719,2.21863137550334));
#10978=CARTESIAN_POINT('Ctrl Pts',(2.38490822912943,55.4942251910797,2.21958486623663));
#10979=CARTESIAN_POINT('Ctrl Pts',(2.97318977758978,54.9684279139246,2.22195490734826));
#10980=CARTESIAN_POINT('Ctrl Pts',(0.772591931467188,55.7451294709179,2.47780062126727));
#10981=CARTESIAN_POINT('Ctrl Pts',(1.59934858958684,55.7362874995129,2.47769305658212));
#10982=CARTESIAN_POINT('Ctrl Pts',(2.38240222522867,55.4903197198984,2.47922620961122));
#10983=CARTESIAN_POINT('Ctrl Pts',(2.97156409628618,54.9665637470307,2.48298719598219));
#10984=CARTESIAN_POINT('',(2.79999999922762,55.7079964370423,2.));
#10985=CARTESIAN_POINT('Ctrl Pts',(0.780904059217545,56.2445672509427,2.));
#10986=CARTESIAN_POINT('Ctrl Pts',(1.4829815941067,56.2396747371019,2.));
#10987=CARTESIAN_POINT('Ctrl Pts',(2.19625600357399,56.0688177741594,2.));
#10988=CARTESIAN_POINT('Ctrl Pts',(2.80042852309129,55.7087104005398,2.));
#10989=CARTESIAN_POINT('',(2.8,55.359994587709,2.09491355855719));
#10990=CARTESIAN_POINT('Ctrl Pts',(2.79999999999999,55.7079964361128,2.));
#10991=CARTESIAN_POINT('Ctrl Pts',(2.79999999999999,55.659531184896,2.));
#10992=CARTESIAN_POINT('Ctrl Pts',(2.79999999998947,55.6110538105124,2.00517381305814));
#10993=CARTESIAN_POINT('Ctrl Pts',(2.79999999998947,55.5164155335608,2.02544396016552));
#10994=CARTESIAN_POINT('Ctrl Pts',(2.79999999999996,55.4701792356063,2.04052661685823));
#10995=CARTESIAN_POINT('Ctrl Pts',(2.79999999999996,55.4034746461591,2.07062671510575));
#10996=CARTESIAN_POINT('Ctrl Pts',(2.79999999999998,55.3813520773532,2.08214461021052));
#10997=CARTESIAN_POINT('Ctrl Pts',(2.79999999999998,55.359994587709,2.0949135585572));
#10998=CARTESIAN_POINT('Ctrl Pts',(2.97156409628599,54.9665637470306,2.48298719598933));
#10999=CARTESIAN_POINT('Ctrl Pts',(2.97106588998616,54.9670303350916,2.48227619063589));
#11000=CARTESIAN_POINT('Ctrl Pts',(2.97056853930023,54.9674978995121,2.48156522401649));
#11001=CARTESIAN_POINT('Ctrl Pts',(2.91166555208744,55.0230844632908,2.39722260558573));
#11002=CARTESIAN_POINT('Ctrl Pts',(2.8635616296325,55.0931658791427,2.31195530150665));
#11003=CARTESIAN_POINT('Ctrl Pts',(2.81284170698683,55.2301922759081,2.18416468374735));
#11004=CARTESIAN_POINT('Ctrl Pts',(2.8,55.2927619192075,2.13510978412522));
#11005=CARTESIAN_POINT('Ctrl Pts',(2.8,55.359994587709,2.09491355855718));
#11006=CARTESIAN_POINT('Origin',(1.15,56.75,2.));
#11007=CARTESIAN_POINT('',(2.80000000000027,57.2719725101481,2.));
#11008=CARTESIAN_POINT('Ctrl Pts',(2.80000000335065,57.271971836207,1.999973299767));
#11009=CARTESIAN_POINT('Ctrl Pts',(2.0202116745349,57.268095273033,1.99997329939139));
#11010=CARTESIAN_POINT('Ctrl Pts',(1.2401748212868,57.1446587362222,1.99997332725321));
#11011=CARTESIAN_POINT('Ctrl Pts',(0.499674955335824,56.8988024033561,1.99997341417823));
#11012=CARTESIAN_POINT('',(2.8,55.,2.));
#11013=CARTESIAN_POINT('Ctrl Pts',(5.00202436963841,49.989878151808,-2.22044604925031E-15));
#11014=CARTESIAN_POINT('Ctrl Pts',(5.00202436963841,49.989878151808,7.4781340831248));
#11015=CARTESIAN_POINT('Ctrl Pts',(5.00202436963841,46.5824238544682,22.4338465954497));
#11016=CARTESIAN_POINT('Ctrl Pts',(5.00202436963841,33.8244208904356,38.4164015488718));
#11017=CARTESIAN_POINT('Ctrl Pts',(5.00202436963841,18.5365493188635,47.2330284289778));
#11018=CARTESIAN_POINT('Ctrl Pts',(5.0020243696384,3.7921966348747,50.6001244586861));
#11019=CARTESIAN_POINT('Ctrl Pts',(5.0020243696384,-11.291748863452,49.4699224532078));
#11020=CARTESIAN_POINT('Ctrl Pts',(5.0020243696384,-25.3711805123871,43.9436357584199));
#11021=CARTESIAN_POINT('Ctrl Pts',(5.0020243696384,-37.1965663489811,34.5127794693327));
#11022=CARTESIAN_POINT('Ctrl Pts',(5.0020243696384,-45.716722944586,22.0157078788456));
#11023=CARTESIAN_POINT('Ctrl Pts',(5.00202436963841,-50.1757699818694,7.56216622012327));
#11024=CARTESIAN_POINT('Ctrl Pts',(5.00202436963842,-50.1744084161316,-7.56296809855995));
#11025=CARTESIAN_POINT('Ctrl Pts',(5.00202436963841,-45.7172849551752,-22.0169942557115));
#11026=CARTESIAN_POINT('Ctrl Pts',(5.00202436963841,-37.1958926535692,-34.5136103597803));
#11027=CARTESIAN_POINT('Ctrl Pts',(5.00202436963841,-25.3703376743228,-43.9440907894173));
#11028=CARTESIAN_POINT('Ctrl Pts',(5.0020243696384,-13.6368192719076,-48.5482363043008));
#11029=CARTESIAN_POINT('Ctrl Pts',(5.0020243696384,-3.74898459555225,-50.0354870397972));
#11030=CARTESIAN_POINT('Ctrl Pts',(5.0020243696384,6.25101355451332,-50.0394425322242));
#11031=CARTESIAN_POINT('Ctrl Pts',(5.00202436963841,18.5371244083236,-47.2318221291753));
#11032=CARTESIAN_POINT('Ctrl Pts',(5.0020243696384,33.8251226771782,-38.416165850227));
#11033=CARTESIAN_POINT('Ctrl Pts',(5.00202436963841,46.5828909425141,-22.4323095026409));
#11034=CARTESIAN_POINT('Ctrl Pts',(5.0020243696384,49.989878151808,-7.47813408312484));
#11035=CARTESIAN_POINT('Ctrl Pts',(5.0020243696384,49.989878151808,-2.44249065417534E-14));
#11036=CARTESIAN_POINT('Ctrl Pts',(5.00068205190813,49.9965897404593,-2.22119182093928E-15));
#11037=CARTESIAN_POINT('Ctrl Pts',(5.00068205190813,49.9965897404593,7.47913808945617));
#11038=CARTESIAN_POINT('Ctrl Pts',(5.00068205190813,46.588677961852,22.4368585402377));
#11039=CARTESIAN_POINT('Ctrl Pts',(5.00068205190813,33.8289621217263,38.42155929466));
#11040=CARTESIAN_POINT('Ctrl Pts',(5.00068205190813,18.5390380165073,47.2393698858715));
#11041=CARTESIAN_POINT('Ctrl Pts',(5.00068205190813,3.79270577122635,50.6069179783561));
#11042=CARTESIAN_POINT('Ctrl Pts',(5.00068205190813,-11.2932648818068,49.4765642331324));
#11043=CARTESIAN_POINT('Ctrl Pts',(5.00068205190813,-25.3745868205016,43.9495355848871));
#11044=CARTESIAN_POINT('Ctrl Pts',(5.00068205190813,-37.2015603209659,34.5174131189366));
#11045=CARTESIAN_POINT('Ctrl Pts',(5.00068205190813,-45.7228608238853,22.0186636847214));
#11046=CARTESIAN_POINT('Ctrl Pts',(5.00068205190814,-50.1825065281432,7.5631815085935));
#11047=CARTESIAN_POINT('Ctrl Pts',(5.00068205190814,-50.1811447796148,-7.5639834947219));
#11048=CARTESIAN_POINT('Ctrl Pts',(5.00068205190813,-45.7234229099287,-22.019950234269));
#11049=CARTESIAN_POINT('Ctrl Pts',(5.00068205190813,-37.2008865351074,-34.5182441209412));
#11050=CARTESIAN_POINT('Ctrl Pts',(5.00068205190814,-25.3737438692996,-43.9499906769628));
#11051=CARTESIAN_POINT('Ctrl Pts',(5.00068205190813,-13.6386501369243,-48.5547543396211));
#11052=CARTESIAN_POINT('Ctrl Pts',(5.00068205190813,-3.74948793029787,-50.0422047518384));
#11053=CARTESIAN_POINT('Ctrl Pts',(5.00068205190813,6.25185280903391,-50.0461607753142));
#11054=CARTESIAN_POINT('Ctrl Pts',(5.00068205190813,18.5396131832233,-47.2381634241137));
#11055=CARTESIAN_POINT('Ctrl Pts',(5.00068205190814,33.8296640026347,-38.4213235643879));
#11056=CARTESIAN_POINT('Ctrl Pts',(5.00068205190814,46.5891451126407,-22.4353212410508));
#11057=CARTESIAN_POINT('Ctrl Pts',(5.00068205190813,49.9965897404593,-7.47913808945619));
#11058=CARTESIAN_POINT('Ctrl Pts',(5.00068205190813,49.9965897404594,-2.4429070022793E-14));
#11059=CARTESIAN_POINT('Ctrl Pts',(4.99947756609878,50.003328895164,-2.22256181089655E-15));
#11060=CARTESIAN_POINT('Ctrl Pts',(4.99947756609878,50.003328895164,7.48014621959278));
#11061=CARTESIAN_POINT('Ctrl Pts',(4.99947756609879,46.5949577563329,22.4398828557256));
#11062=CARTESIAN_POINT('Ctrl Pts',(4.99947756609878,33.8335220049191,38.4267382245323));
#11063=CARTESIAN_POINT('Ctrl Pts',(4.99947756609878,18.5415369358535,47.2457373886046));
#11064=CARTESIAN_POINT('Ctrl Pts',(4.99947756609878,3.79321699871334,50.6137394006006));
#11065=CARTESIAN_POINT('Ctrl Pts',(4.99947756609877,-11.2947871268155,49.4832332924101));
#11066=CARTESIAN_POINT('Ctrl Pts',(4.99947756609878,-25.3780071191065,43.9554596433293));
#11067=CARTESIAN_POINT('Ctrl Pts',(4.99947756609878,-37.206574804386,34.5220658000138));
#11068=CARTESIAN_POINT('Ctrl Pts',(4.99947756609877,-45.729023912893,22.0216316307696));
#11069=CARTESIAN_POINT('Ctrl Pts',(4.99947756609878,-50.1892707429977,7.56420096713228));
#11070=CARTESIAN_POINT('Ctrl Pts',(4.99947756609879,-50.1879088109157,-7.56500306136105));
#11071=CARTESIAN_POINT('Ctrl Pts',(4.99947756609878,-45.7295860747013,-22.0229183537352));
#11072=CARTESIAN_POINT('Ctrl Pts',(4.99947756609878,-37.2059009277063,-34.522896914031));
#11073=CARTESIAN_POINT('Ctrl Pts',(4.99947756609878,-25.3771640542804,-43.9559147967486));
#11074=CARTESIAN_POINT('Ctrl Pts',(4.99947756609877,-13.6404885217781,-48.561299146034));
#11075=CARTESIAN_POINT('Ctrl Pts',(4.99947756609878,-3.74999333235333,-50.0489500550953));
#11076=CARTESIAN_POINT('Ctrl Pts',(4.99947756609877,6.25269551057625,-50.0529066118129));
#11077=CARTESIAN_POINT('Ctrl Pts',(4.99947756609878,18.5421121800959,-47.2445307642251));
#11078=CARTESIAN_POINT('Ctrl Pts',(4.99947756609877,33.8342239804377,-38.426502462485));
#11079=CARTESIAN_POINT('Ctrl Pts',(4.99947756609879,46.5954249700887,-22.438345349323));
#11080=CARTESIAN_POINT('Ctrl Pts',(4.99947756609877,50.003328895164,-7.48014621959283));
#11081=CARTESIAN_POINT('Ctrl Pts',(4.99947756609877,50.003328895164,-2.44326092853315E-14));
#11082=CARTESIAN_POINT('Ctrl Pts',(4.99841192763649,50.010089934565,-2.22455486416984E-15));
#11083=CARTESIAN_POINT('Ctrl Pts',(4.99841192763649,50.010089934565,7.48115762363149));
#11084=CARTESIAN_POINT('Ctrl Pts',(4.9984119276365,46.6012579438089,22.4429169923092));
#11085=CARTESIAN_POINT('Ctrl Pts',(4.99841192763649,33.8380966958625,38.4319339724568));
#11086=CARTESIAN_POINT('Ctrl Pts',(4.99841192763649,18.5440439702159,47.2521255691362));
#11087=CARTESIAN_POINT('Ctrl Pts',(4.99841192763649,3.7937298863526,50.6205829747067));
#11088=CARTESIAN_POINT('Ctrl Pts',(4.99841192763649,-11.2963143151676,49.4899240087747));
#11089=CARTESIAN_POINT('Ctrl Pts',(4.99841192763649,-25.3814385247641,43.9614029395442));
#11090=CARTESIAN_POINT('Ctrl Pts',(4.99841192763649,-37.2116055718427,34.5267335901821));
#11091=CARTESIAN_POINT('Ctrl Pts',(4.99841192763649,-45.7352070158957,22.0246092149029));
#11092=CARTESIAN_POINT('Ctrl Pts',(4.9984119276365,-50.1960569239472,7.56522373629383));
#11093=CARTESIAN_POINT('Ctrl Pts',(4.9984119276365,-50.1946948077045,-7.566025938944));
#11094=CARTESIAN_POINT('Ctrl Pts',(4.99841192763649,-45.7357692537155,-22.0258961118735));
#11095=CARTESIAN_POINT('Ctrl Pts',(4.99841192763649,-37.210931604044,-34.5275648165732));
#11096=CARTESIAN_POINT('Ctrl Pts',(4.9984119276365,-25.3805953459256,-43.9618581545187));
#11097=CARTESIAN_POINT('Ctrl Pts',(4.99841192763649,-13.6423328766374,-48.5678652060244));
#11098=CARTESIAN_POINT('Ctrl Pts',(4.99841192763649,-3.75050037564627,-50.055717263026));
#11099=CARTESIAN_POINT('Ctrl Pts',(4.99841192763649,6.25354094871083,-50.0596743547279));
#11100=CARTESIAN_POINT('Ctrl Pts',(4.9984119276365,18.5446192921948,-47.2509187816055));
#11101=CARTESIAN_POINT('Ctrl Pts',(4.99841192763649,33.8387987663498,-38.4316981785149));
#11102=CARTESIAN_POINT('Ctrl Pts',(4.9984119276365,46.6017252207067,-22.4413792780267));
#11103=CARTESIAN_POINT('Ctrl Pts',(4.99841192763649,50.010089934565,-7.48115762363152));
#11104=CARTESIAN_POINT('Ctrl Pts',(4.99841192763649,50.0100899345651,-2.44355213456396E-14));
#11105=CARTESIAN_POINT('',(5.00202436963841,49.989878151808,-2.22044604925031E-15));
#11106=CARTESIAN_POINT('Origin',(5.49231470748387,50.0879362193771,-4.44089209850063E-15));
#11107=CARTESIAN_POINT('',(5.00202436963841,-49.9893356667678,9.68104724163865E-7));
#11108=CARTESIAN_POINT('Ctrl Pts',(5.00202436963841,49.989878151808,-2.22044604925031E-15));
#11109=CARTESIAN_POINT('Ctrl Pts',(5.00202436963841,49.989878151808,7.4781340831248));
#11110=CARTESIAN_POINT('Ctrl Pts',(5.00202436963841,46.5824238544682,22.4338465954497));
#11111=CARTESIAN_POINT('Ctrl Pts',(5.00202436963841,33.8244208904356,38.4164015488718));
#11112=CARTESIAN_POINT('Ctrl Pts',(5.00202436963841,18.5365493188635,47.2330284289778));
#11113=CARTESIAN_POINT('Ctrl Pts',(5.0020243696384,3.7921966348747,50.6001244586861));
#11114=CARTESIAN_POINT('Ctrl Pts',(5.0020243696384,-11.291748863452,49.4699224532078));
#11115=CARTESIAN_POINT('Ctrl Pts',(5.0020243696384,-25.3711805123871,43.9436357584199));
#11116=CARTESIAN_POINT('Ctrl Pts',(5.0020243696384,-37.1965663489811,34.5127794693327));
#11117=CARTESIAN_POINT('Ctrl Pts',(5.0020243696384,-45.716722944586,22.0157078788456));
#11118=CARTESIAN_POINT('Ctrl Pts',(5.00202436963841,-49.4325545339432,9.9712225382536));
#11119=CARTESIAN_POINT('Ctrl Pts',(5.00202436963841,-49.9894453154963,2.49274641922705));
#11120=CARTESIAN_POINT('Ctrl Pts',(5.00202436963841,-49.9893356667678,9.68104723747532E-7));
#11121=CARTESIAN_POINT('Ctrl Pts',(5.00202436963841,-49.9893356667678,9.68104723747532E-7));
#11122=CARTESIAN_POINT('Ctrl Pts',(5.00202436963841,-49.9892260059575,-2.49301915037777));
#11123=CARTESIAN_POINT('Ctrl Pts',(5.00202436963841,-49.4315954300228,-9.9718397452934));
#11124=CARTESIAN_POINT('Ctrl Pts',(5.00202436963841,-45.7172849551752,-22.0169942557115));
#11125=CARTESIAN_POINT('Ctrl Pts',(5.00202436963841,-37.1958926535692,-34.5136103597803));
#11126=CARTESIAN_POINT('Ctrl Pts',(5.00202436963841,-25.3703376743228,-43.9440907894173));
#11127=CARTESIAN_POINT('Ctrl Pts',(5.0020243696384,-13.6368192719076,-48.5482363043008));
#11128=CARTESIAN_POINT('Ctrl Pts',(5.0020243696384,-3.74898459555225,-50.0354870397972));
#11129=CARTESIAN_POINT('Ctrl Pts',(5.0020243696384,6.25101355451332,-50.0394425322242));
#11130=CARTESIAN_POINT('Ctrl Pts',(5.00202436963841,18.5371244083236,-47.2318221291753));
#11131=CARTESIAN_POINT('Ctrl Pts',(5.0020243696384,33.8251226771782,-38.416165850227));
#11132=CARTESIAN_POINT('Ctrl Pts',(5.00202436963841,46.5828909425141,-22.4323095026409));
#11133=CARTESIAN_POINT('Ctrl Pts',(5.0020243696384,49.989878151808,-7.47813408312484));
#11134=CARTESIAN_POINT('Ctrl Pts',(5.0020243696384,49.989878151808,-2.44249065417534E-14));
#11135=CARTESIAN_POINT('Origin',(8.,0.,0.));
#11136=CARTESIAN_POINT('',(11.,-20.,-2.44929359829471E-15));
#11137=CARTESIAN_POINT('Origin',(11.,0.,0.));
#11138=CARTESIAN_POINT('',(8.,-35.,-4.28626379701574E-15));
#11139=CARTESIAN_POINT('Origin',(5.5,0.,0.));
#11140=CARTESIAN_POINT('',(5.5,-1.46957615897682E-15,12.));
#11141=CARTESIAN_POINT('',(5.5,-12.,-1.46957615897682E-15));
#11142=CARTESIAN_POINT('Origin',(5.5,0.,0.));
#11143=CARTESIAN_POINT('Origin',(5.5,0.,0.));
#11144=CARTESIAN_POINT('',(5.,-1.40834381901946E-15,11.5));
#11145=CARTESIAN_POINT('Origin',(5.5,-1.40834381901946E-15,11.5));
#11146=CARTESIAN_POINT('Origin',(5.,0.,0.));
#11147=CARTESIAN_POINT('Origin',(5.,12.,0.));
#11148=CARTESIAN_POINT('',(5.,7.8995253021938,3.));
#11149=CARTESIAN_POINT('',(5.,10.74,3.));
#11150=CARTESIAN_POINT('',(5.,10.31,3.));
#11151=CARTESIAN_POINT('',(5.,7.8995253021938,-3.));
#11152=CARTESIAN_POINT('Origin',(5.,0.,0.));
#11153=CARTESIAN_POINT('',(5.,10.74,-3.));
#11154=CARTESIAN_POINT('',(5.,10.31,-3.));
#11155=CARTESIAN_POINT('',(5.,10.74,0.));
#11156=CARTESIAN_POINT('Origin',(8.,0.,0.));
#11157=CARTESIAN_POINT('',(11.,-12.,-1.46957615897682E-15));
#11158=CARTESIAN_POINT('Origin',(11.,0.,0.));
#11159=CARTESIAN_POINT('',(8.,-12.,-1.46957615897682E-15));
#11160=CARTESIAN_POINT('Origin',(5.5,10.74,0.));
#11161=CARTESIAN_POINT('',(5.5,10.24,-2.5));
#11162=CARTESIAN_POINT('Origin',(5.5,10.74,-3.));
#11163=CARTESIAN_POINT('',(5.5,10.24,2.5));
#11164=CARTESIAN_POINT('',(5.5,10.24,0.));
#11165=CARTESIAN_POINT('Origin',(5.5,10.74,3.));
#11166=CARTESIAN_POINT('Origin',(5.5,10.31,3.));
#11167=CARTESIAN_POINT('',(5.5,7.8995253021938,2.5));
#11168=CARTESIAN_POINT('',(5.5,10.31,2.5));
#11169=CARTESIAN_POINT('Origin',(5.5,7.8995253021938,3.));
#11170=CARTESIAN_POINT('Origin',(5.5,7.8995253021938,3.));
#11171=CARTESIAN_POINT('',(5.5,7.43209776951961,2.82248520710059));
#11172=CARTESIAN_POINT('Origin',(5.5,7.8995253021938,3.));
#11173=CARTESIAN_POINT('Origin',(5.5,7.8995253021938,3.));
#11174=CARTESIAN_POINT('Origin',(5.5,0.,0.));
#11175=CARTESIAN_POINT('',(5.5,7.43209776951961,-2.82248520710059));
#11176=CARTESIAN_POINT('Origin',(5.5,0.,0.));
#11177=CARTESIAN_POINT('Origin',(5.5,7.8995253021938,-3.));
#11178=CARTESIAN_POINT('Origin',(9.,7.8995253021938,3.));
#11179=CARTESIAN_POINT('',(12.5,7.8995253021938,2.5));
#11180=CARTESIAN_POINT('',(9.,7.8995253021938,2.5));
#11181=CARTESIAN_POINT('',(12.5,7.43209776951961,2.82248520710059));
#11182=CARTESIAN_POINT('Origin',(12.5,7.8995253021938,3.));
#11183=CARTESIAN_POINT('',(9.,7.43209776951961,2.82248520710059));
#11184=CARTESIAN_POINT('Origin',(9.,8.62,2.5));
#11185=CARTESIAN_POINT('',(12.5,10.24,2.5));
#11186=CARTESIAN_POINT('',(14.,10.24,2.5));
#11187=CARTESIAN_POINT('',(12.5,8.285,2.5));
#11188=CARTESIAN_POINT('Origin',(14.,10.24,0.));
#11189=CARTESIAN_POINT('',(12.5,10.24,-2.5));
#11190=CARTESIAN_POINT('',(14.,10.24,-2.5));
#11191=CARTESIAN_POINT('',(12.5,10.24,0.));
#11192=CARTESIAN_POINT('Origin',(12.5,10.74,0.));
#11193=CARTESIAN_POINT('',(13.,10.74,-3.));
#11194=CARTESIAN_POINT('Origin',(12.5,10.74,-3.));
#11195=CARTESIAN_POINT('',(13.,10.74,3.));
#11196=CARTESIAN_POINT('',(13.,10.74,0.));
#11197=CARTESIAN_POINT('Origin',(12.5,10.74,3.));
#11198=CARTESIAN_POINT('Origin',(12.5,7.8995253021938,3.));
#11199=CARTESIAN_POINT('',(13.,7.8995253021938,3.));
#11200=CARTESIAN_POINT('Origin',(12.5,7.8995253021938,3.));
#11201=CARTESIAN_POINT('Origin',(12.5,7.8995253021938,3.));
#11202=CARTESIAN_POINT('Origin',(12.5,8.285,3.));
#11203=CARTESIAN_POINT('',(13.,8.285,3.));
#11204=CARTESIAN_POINT('Origin',(12.5,0.,0.));
#11205=CARTESIAN_POINT('',(13.,7.8995253021938,-3.));
#11206=CARTESIAN_POINT('Origin',(13.,0.,0.));
#11207=CARTESIAN_POINT('',(12.5,7.43209776951961,-2.82248520710059));
#11208=CARTESIAN_POINT('Origin',(12.5,7.8995253021938,-3.));
#11209=CARTESIAN_POINT('Origin',(12.5,0.,0.));
#11210=CARTESIAN_POINT('Origin',(12.5,0.,0.));
#11211=CARTESIAN_POINT('',(13.,-2.4440003129991E-15,19.9567770454363));
#11212=CARTESIAN_POINT('Origin',(13.,0.,0.));
#11213=CARTESIAN_POINT('',(12.9925825347358,-2.45450835807069E-15,20.0425817450355));
#11214=CARTESIAN_POINT('Origin',(12.5,-2.4440003129991E-15,19.9567770454363));
#11215=CARTESIAN_POINT('',(12.9925825347358,-20.0425817450355,-2.45450835807069E-15));
#11216=CARTESIAN_POINT('Origin',(12.9925825347358,0.,-3.06813544758836E-15));
#11217=CARTESIAN_POINT('Origin',(12.9925825347358,0.,-3.06813544758836E-15));
#11218=CARTESIAN_POINT('Origin',(13.,7.95,0.));
#11219=CARTESIAN_POINT('',(13.,8.285,-3.));
#11220=CARTESIAN_POINT('Origin',(10.3,0.,0.));
#11221=CARTESIAN_POINT('',(7.6,-51.,-6.2456986756515E-15));
#11222=CARTESIAN_POINT('',(10.3,-35.5,-4.3474961369731E-15));
#11223=CARTESIAN_POINT('',(7.6,51.,0.));
#11224=CARTESIAN_POINT('Origin',(7.6,0.,0.));
#11225=CARTESIAN_POINT('Origin',(7.6,0.,0.));
#11226=CARTESIAN_POINT('Origin',(5.5,7.8995253021938,-3.));
#11227=CARTESIAN_POINT('',(5.5,7.8995253021938,-2.5));
#11228=CARTESIAN_POINT('Origin',(5.5,7.8995253021938,-3.));
#11229=CARTESIAN_POINT('Origin',(5.5,7.8995253021938,-3.));
#11230=CARTESIAN_POINT('Origin',(5.5,10.31,-3.));
#11231=CARTESIAN_POINT('',(5.5,10.31,-2.5));
#11232=CARTESIAN_POINT('Origin',(9.,7.8995253021938,-3.));
#11233=CARTESIAN_POINT('',(12.5,7.8995253021938,-2.5));
#11234=CARTESIAN_POINT('Origin',(12.5,7.8995253021938,-3.));
#11235=CARTESIAN_POINT('',(9.,7.8995253021938,-2.5));
#11236=CARTESIAN_POINT('',(9.,7.43209776951961,-2.82248520710059));
#11237=CARTESIAN_POINT('Origin',(12.5,7.8995253021938,-3.));
#11238=CARTESIAN_POINT('Origin',(12.5,7.8995253021938,-3.));
#11239=CARTESIAN_POINT('Origin',(9.,8.62,-2.5));
#11240=CARTESIAN_POINT('',(12.5,8.285,-2.5));
#11241=CARTESIAN_POINT('Origin',(12.5,8.285,-3.));
#11242=CARTESIAN_POINT('Origin',(9.,0.,0.));
#11243=CARTESIAN_POINT('Ctrl Pts',(0.,56.8978458123625,2.49999999999978));
#11244=CARTESIAN_POINT('Ctrl Pts',(0.,56.5290913566253,10.8925336660656));
#11245=CARTESIAN_POINT('Ctrl Pts',(0.,52.0239399392849,27.5104427981014));
#11246=CARTESIAN_POINT('Ctrl Pts',(0.,37.0895128901808,44.9505513524534));
#11247=CARTESIAN_POINT('Ctrl Pts',(0.,19.6413066333793,54.3407718417784));
#11248=CARTESIAN_POINT('Ctrl Pts',(0.,2.98972976337264,57.7126473424414));
#11249=CARTESIAN_POINT('Ctrl Pts',(0.,-13.9100795010715,56.0762889490297));
#11250=CARTESIAN_POINT('Ctrl Pts',(0.,-34.8726547481504,47.4775611101652));
#11251=CARTESIAN_POINT('Ctrl Pts',(0.,-48.6578954952714,32.3601597542925));
#11252=CARTESIAN_POINT('Ctrl Pts',(0.,-54.6754985459398,16.615078371656));
#11253=CARTESIAN_POINT('Ctrl Pts',(0.,-58.4322800872165,0.182637285551057));
#11254=CARTESIAN_POINT('Ctrl Pts',(0.,-55.3972091422166,-20.0478023034309));
#11255=CARTESIAN_POINT('Ctrl Pts',(0.,-42.7587268357465,-38.8566003856648));
#11256=CARTESIAN_POINT('Ctrl Pts',(0.,-29.6277979733952,-49.6176180623964));
#11257=CARTESIAN_POINT('Ctrl Pts',(0.,-13.9134722149986,-56.083084294608));
#11258=CARTESIAN_POINT('Ctrl Pts',(0.,2.99163137042858,-57.710045079662));
#11259=CARTESIAN_POINT('Ctrl Pts',(0.,19.6409629692718,-54.3421091676748));
#11260=CARTESIAN_POINT('Ctrl Pts',(0.,37.0902013849514,-44.9493511994273));
#11261=CARTESIAN_POINT('Ctrl Pts',(0.,52.0238383479187,-27.5106172571882));
#11262=CARTESIAN_POINT('Ctrl Pts',(0.,56.5290913566252,-10.8925336660656));
#11263=CARTESIAN_POINT('Ctrl Pts',(0.,56.8978458123625,-2.49999999999977));
#11264=CARTESIAN_POINT('Ctrl Pts',(0.,57.001373876214,2.50454885691929));
#11265=CARTESIAN_POINT('Ctrl Pts',(-1.63742030236312E-19,56.6319480624753,
10.9123620526042));
#11266=CARTESIAN_POINT('Ctrl Pts',(9.48249132196878E-20,52.1186000182248,
27.5604934111569));
#11267=CARTESIAN_POINT('Ctrl Pts',(-1.19995263848322E-19,37.1569994229608,
45.0323427370933));
#11268=CARTESIAN_POINT('Ctrl Pts',(1.23050933331286E-19,19.6770452908852,
54.4396466559896));
#11269=CARTESIAN_POINT('Ctrl Pts',(-1.44052426172425E-19,2.9951686864826,
57.8176582375029));
#11270=CARTESIAN_POINT('Ctrl Pts',(3.14735156619693E-19,-13.935388031018,
56.1783232228821));
#11271=CARTESIAN_POINT('Ctrl Pts',(-6.67633563883309E-19,-34.9361090552895,
47.5639470777454));
#11272=CARTESIAN_POINT('Ctrl Pts',(1.58766279766169E-18,-48.746429713773,
32.4190424283386));
#11273=CARTESIAN_POINT('Ctrl Pts',(-1.26927833601234E-18,-54.774983220983,
16.645310295907));
#11274=CARTESIAN_POINT('Ctrl Pts',(4.57103728577927E-18,-58.5386002359852,
0.182968458669554));
#11275=CARTESIAN_POINT('Ctrl Pts',(-9.06026943189087E-18,-55.4980072978672,
-20.0842792997109));
#11276=CARTESIAN_POINT('Ctrl Pts',(1.1238606803883E-17,-42.8365283395576,
-38.9273017012347));
#11277=CARTESIAN_POINT('Ctrl Pts',(-3.02518942121921E-17,-29.68170664745,
-49.7079003853428));
#11278=CARTESIAN_POINT('Ctrl Pts',(1.07915148805084E-16,-13.9387883568906,
-56.1851293477377));
#11279=CARTESIAN_POINT('Ctrl Pts',(-2.95307104319226E-18,2.99707413713518,
-57.8150521907767));
#11280=CARTESIAN_POINT('Ctrl Pts',(2.05765094998786E-16,19.6767005375821,
-54.4409860649289));
#11281=CARTESIAN_POINT('Ctrl Pts',(-1.25774157565186E-16,37.1576897427545,
-45.0311405989928));
#11282=CARTESIAN_POINT('Ctrl Pts',(7.30652087057546E-17,52.1184978807484,
-27.5606680742516));
#11283=CARTESIAN_POINT('Ctrl Pts',(1.96124639940372E-19,56.6319480624753,
-10.9123620526041));
#11284=CARTESIAN_POINT('Ctrl Pts',(0.,57.001373876214,-2.50454885691928));
#11285=CARTESIAN_POINT('Ctrl Pts',(0.0667333574462435,57.2080172044309,
2.5136284330116));
#11286=CARTESIAN_POINT('Ctrl Pts',(0.0667333574462435,56.8372529234427,
10.9519039899706));
#11287=CARTESIAN_POINT('Ctrl Pts',(0.0667333574462479,52.3075415566464,
27.6604182942792));
#11288=CARTESIAN_POINT('Ctrl Pts',(0.066733357446241,37.2917010899539,45.1955916525164));
#11289=CARTESIAN_POINT('Ctrl Pts',(0.0667333574462441,19.7483782666853,
54.6370042126952));
#11290=CARTESIAN_POINT('Ctrl Pts',(0.066733357446246,3.00602891262606,58.0272602571566));
#11291=CARTESIAN_POINT('Ctrl Pts',(0.0667333574462456,-13.9859099881671,
56.3819806617786));
#11292=CARTESIAN_POINT('Ctrl Pts',(0.0667333574462422,-35.062756586454,
47.7363804977705));
#11293=CARTESIAN_POINT('Ctrl Pts',(0.066733357446249,-48.9231487449615,
32.5365650856458));
#11294=CARTESIAN_POINT('Ctrl Pts',(0.0667333574462432,-54.9735548269809,
16.7056532862401));
#11295=CARTESIAN_POINT('Ctrl Pts',(0.0667333574462437,-58.7508161372197,
0.183634051074929));
#11296=CARTESIAN_POINT('Ctrl Pts',(0.0667333574462451,-55.6991994401982,
-20.1570911918775));
#11297=CARTESIAN_POINT('Ctrl Pts',(0.0667333574462445,-42.991820442108,
-39.0684221465814));
#11298=CARTESIAN_POINT('Ctrl Pts',(0.0667333574462468,-29.789310528299,
-49.8881012725558));
#11299=CARTESIAN_POINT('Ctrl Pts',(0.0667333574462466,-13.9893197604443,
-56.3888146340892));
#11300=CARTESIAN_POINT('Ctrl Pts',(0.0667333574462478,3.00794050308572,
-58.0246428589159));
#11301=CARTESIAN_POINT('Ctrl Pts',(0.0667333574462471,19.7480331923249,
-54.6383491786078));
#11302=CARTESIAN_POINT('Ctrl Pts',(0.066733357446242,37.2923927665473,-45.1943847586508));
#11303=CARTESIAN_POINT('Ctrl Pts',(0.0667333574462439,52.3074397721863,
-27.6605938176656));
#11304=CARTESIAN_POINT('Ctrl Pts',(0.0667333574462471,56.8372529234427,
-10.9519039899706));
#11305=CARTESIAN_POINT('Ctrl Pts',(0.0667333574462471,57.2080172044309,
-2.51362843301159));
#11306=CARTESIAN_POINT('Ctrl Pts',(0.241146694675275,57.3375734782873,2.51932092769249));
#11307=CARTESIAN_POINT('Ctrl Pts',(0.241146694675275,56.9659668116783,10.9767684555204));
#11308=CARTESIAN_POINT('Ctrl Pts',(0.241146694675289,52.4260020076026,27.7230191395092));
#11309=CARTESIAN_POINT('Ctrl Pts',(0.241146694675268,37.3761578444925,45.2979573924083));
#11310=CARTESIAN_POINT('Ctrl Pts',(0.241146694675277,19.7931046748997,54.7607342556246));
#11311=CARTESIAN_POINT('Ctrl Pts',(0.241146694675283,3.01282945138884,58.1586736724148));
#11312=CARTESIAN_POINT('Ctrl Pts',(0.241146694675282,-14.0175731085778,
56.5096736677099));
#11313=CARTESIAN_POINT('Ctrl Pts',(0.241146694675271,-35.1421755770565,
47.8444764887727));
#11314=CARTESIAN_POINT('Ctrl Pts',(0.241146694675293,-49.0339363965306,
32.6102628457984));
#11315=CARTESIAN_POINT('Ctrl Pts',(0.241146694675275,-55.0980526755376,
16.7434863298973));
#11316=CARTESIAN_POINT('Ctrl Pts',(0.241146694675276,-58.8838671210771,
0.184041977005384));
#11317=CARTESIAN_POINT('Ctrl Pts',(0.241146694675281,-55.825342686821,-20.2027341799597));
#11318=CARTESIAN_POINT('Ctrl Pts',(0.241146694675279,-43.0891831640078,
-39.1568990246098));
#11319=CARTESIAN_POINT('Ctrl Pts',(0.241146694675286,-29.8567703816805,
-50.0010870444588));
#11320=CARTESIAN_POINT('Ctrl Pts',(0.241146694675285,-14.0210005969976,
-56.516512105534));
#11321=CARTESIAN_POINT('Ctrl Pts',(0.241146694675289,3.01474803516986,-58.1560569525823));
#11322=CARTESIAN_POINT('Ctrl Pts',(0.241146694675286,19.7927555967382,-54.7620798342382));
#11323=CARTESIAN_POINT('Ctrl Pts',(0.241146694675271,37.376855062764,-45.2967491452879));
#11324=CARTESIAN_POINT('Ctrl Pts',(0.241146694675276,52.4258974831749,-27.7231942724782));
#11325=CARTESIAN_POINT('Ctrl Pts',(0.241146694675286,56.9659668116783,-10.9767684555204));
#11326=CARTESIAN_POINT('Ctrl Pts',(0.241146694675286,57.3375734782873,-2.51932092769249));
#11327=CARTESIAN_POINT('Ctrl Pts',(0.339274733856657,57.370852629519,2.52078316017057));
#11328=CARTESIAN_POINT('Ctrl Pts',(0.339274733856657,56.9990326206148,10.9830861748047));
#11329=CARTESIAN_POINT('Ctrl Pts',(0.339274733856675,52.4564286898744,27.7391443737182));
#11330=CARTESIAN_POINT('Ctrl Pts',(0.339274733856648,37.397847805002,45.3242371558628));
#11331=CARTESIAN_POINT('Ctrl Pts',(0.339274733856659,19.8045900020693,54.7925210277751));
#11332=CARTESIAN_POINT('Ctrl Pts',(0.339274733856667,3.01458417638844,58.1924278198806));
#11333=CARTESIAN_POINT('Ctrl Pts',(0.339274733856666,-14.0257176651751,
56.5424659470342));
#11334=CARTESIAN_POINT('Ctrl Pts',(0.339274733856652,-35.162560335835,47.8722546129936));
#11335=CARTESIAN_POINT('Ctrl Pts',(0.33927473385668,-49.062401429532,32.6291783076228));
#11336=CARTESIAN_POINT('Ctrl Pts',(0.339274733856656,-55.130030403419,16.7532039056753));
#11337=CARTESIAN_POINT('Ctrl Pts',(0.339274733856658,-58.9180430616952,
0.184155597534577));
#11338=CARTESIAN_POINT('Ctrl Pts',(0.339274733856665,-55.8577407704635,
-20.2144649779688));
#11339=CARTESIAN_POINT('Ctrl Pts',(0.339274733856663,-43.114191423157,-39.1796255654678));
#11340=CARTESIAN_POINT('Ctrl Pts',(0.339274733856671,-29.8741016817107,
-50.03010242379));
#11341=CARTESIAN_POINT('Ctrl Pts',(0.339274733856671,-14.0291385836291,
-56.5493177841146));
#11342=CARTESIAN_POINT('Ctrl Pts',(0.339274733856675,3.01650159200602,-58.1898039238036));
#11343=CARTESIAN_POINT('Ctrl Pts',(0.339274733856671,19.8042434809913,-54.7938694712148));
#11344=CARTESIAN_POINT('Ctrl Pts',(0.339274733856652,37.3985420234115,-45.3230270256477));
#11345=CARTESIAN_POINT('Ctrl Pts',(0.339274733856658,52.4563262539523,-27.7393202831295));
#11346=CARTESIAN_POINT('Ctrl Pts',(0.339274733856671,56.9990326206148,-10.9830861748047));
#11347=CARTESIAN_POINT('Ctrl Pts',(0.339274733856672,57.370852629519,-2.52078316017056));
#11348=CARTESIAN_POINT('',(0.339274733856678,57.370852629519,-2.52078316017068));
#11349=CARTESIAN_POINT('Origin',(0.499999999999991,56.8978458123625,-2.49999999999977));
#11350=CARTESIAN_POINT('',(0.33927473385663,57.370852629519,2.52078316017068));
#11351=CARTESIAN_POINT('Ctrl Pts',(0.339274733856672,57.370852629519,-2.52078316017056));
#11352=CARTESIAN_POINT('Ctrl Pts',(0.339274733856671,56.9990326206148,-10.9830861748047));
#11353=CARTESIAN_POINT('Ctrl Pts',(0.339274733856658,52.4563262539523,-27.7393202831295));
#11354=CARTESIAN_POINT('Ctrl Pts',(0.339274733856652,37.3985420234115,-45.3230270256477));
#11355=CARTESIAN_POINT('Ctrl Pts',(0.339274733856671,19.8042434809913,-54.7938694712148));
#11356=CARTESIAN_POINT('Ctrl Pts',(0.339274733856675,3.01650159200602,-58.1898039238036));
#11357=CARTESIAN_POINT('Ctrl Pts',(0.339274733856671,-14.0291385836291,
-56.5493177841146));
#11358=CARTESIAN_POINT('Ctrl Pts',(0.339274733856671,-29.8741016817107,
-50.03010242379));
#11359=CARTESIAN_POINT('Ctrl Pts',(0.339274733856663,-43.114191423157,-39.1796255654678));
#11360=CARTESIAN_POINT('Ctrl Pts',(0.339274733856665,-55.8577407704635,
-20.2144649779688));
#11361=CARTESIAN_POINT('Ctrl Pts',(0.339274733856658,-58.9180430616952,
0.184155597534577));
#11362=CARTESIAN_POINT('Ctrl Pts',(0.339274733856656,-55.130030403419,16.7532039056753));
#11363=CARTESIAN_POINT('Ctrl Pts',(0.33927473385668,-49.062401429532,32.6291783076228));
#11364=CARTESIAN_POINT('Ctrl Pts',(0.339274733856652,-35.162560335835,47.8722546129936));
#11365=CARTESIAN_POINT('Ctrl Pts',(0.339274733856666,-14.0257176651751,
56.5424659470342));
#11366=CARTESIAN_POINT('Ctrl Pts',(0.339274733856667,3.01458417638844,58.1924278198806));
#11367=CARTESIAN_POINT('Ctrl Pts',(0.339274733856659,19.8045900020693,54.7925210277751));
#11368=CARTESIAN_POINT('Ctrl Pts',(0.339274733856648,37.397847805002,45.3242371558628));
#11369=CARTESIAN_POINT('Ctrl Pts',(0.339274733856675,52.4564286898744,27.7391443737182));
#11370=CARTESIAN_POINT('Ctrl Pts',(0.339274733856657,56.9990326206148,10.9830861748047));
#11371=CARTESIAN_POINT('Ctrl Pts',(0.339274733856657,57.370852629519,2.52078316017057));
#11372=CARTESIAN_POINT('Origin',(0.499999999999996,56.8978458123625,2.49999999999978));
#11373=CARTESIAN_POINT('Origin',(0.5,57.025,-2.5));
#11374=CARTESIAN_POINT('',(0.500000000000238,56.8978458123627,-2.));
#11375=CARTESIAN_POINT('',(0.5,57.025,-2.));
#11376=CARTESIAN_POINT('Origin',(0.5,56.8978458123627,-2.5));
#11377=CARTESIAN_POINT('Origin',(0.499999999999896,56.8978458123625,-2.50000000000002));
#11378=CARTESIAN_POINT('Origin',(0.499999999999896,56.8978458123625,-2.50000000000002));
#11379=CARTESIAN_POINT('Origin',(0.50000000000006,56.8978458123625,2.5));
#11380=CARTESIAN_POINT('Origin',(0.50000000000006,56.8978458123625,2.5));
#11381=CARTESIAN_POINT('Ctrl Pts',(3.30000000000023,57.2570611822017,2.));
#11382=CARTESIAN_POINT('Ctrl Pts',(2.35587473833117,57.3142929108325,2.));
#11383=CARTESIAN_POINT('Ctrl Pts',(1.39877068709439,57.1962523550954,2.));
#11384=CARTESIAN_POINT('Ctrl Pts',(0.499999999999973,56.8978458123625,2.));
#11385=CARTESIAN_POINT('Ctrl Pts',(3.31887371652615,57.5315882986027,1.99241789689239));
#11386=CARTESIAN_POINT('Ctrl Pts',(2.33276518160034,57.5906485008098,1.99241414329163));
#11387=CARTESIAN_POINT('Ctrl Pts',(1.35243127070208,57.4698597329915,1.99241931647724));
#11388=CARTESIAN_POINT('Ctrl Pts',(0.411584403188821,57.1580487103768,1.99244885315961));
#11389=CARTESIAN_POINT('Ctrl Pts',(3.33560242564919,57.7749152697563,2.24717484796588));
#11390=CARTESIAN_POINT('Ctrl Pts',(2.31227799847597,57.8355775691271,2.24725411917667));
#11391=CARTESIAN_POINT('Ctrl Pts',(1.3113738729421,57.7123824082935,2.24714501562381));
#11392=CARTESIAN_POINT('Ctrl Pts',(0.33317230266513,57.3888117943974,2.24652030369265));
#11393=CARTESIAN_POINT('Ctrl Pts',(3.33426151832809,57.7554111397819,2.52175932309878));
#11394=CARTESIAN_POINT('Ctrl Pts',(2.31390369740501,57.8158698649554,2.52187727319098));
#11395=CARTESIAN_POINT('Ctrl Pts',(1.31472805667249,57.6929865211876,2.52171535509758));
#11396=CARTESIAN_POINT('Ctrl Pts',(0.339274733856594,57.370852629519,2.52078316017079));
#11397=CARTESIAN_POINT('',(3.33426151832784,57.7554111397819,2.5217593230988));
#11398=CARTESIAN_POINT('Ctrl Pts',(0.339274733856594,57.370852629519,2.52078316017079));
#11399=CARTESIAN_POINT('Ctrl Pts',(1.31472805667249,57.6929865211876,2.52171535509758));
#11400=CARTESIAN_POINT('Ctrl Pts',(2.31390369740501,57.8158698649554,2.52187727319098));
#11401=CARTESIAN_POINT('Ctrl Pts',(3.33426151832809,57.7554111397819,2.52175932309878));
#11402=CARTESIAN_POINT('',(2.8,57.2767052616368,2.00002239837059));
#11403=CARTESIAN_POINT('Ctrl Pts',(2.8,57.2767052616368,2.00002239837057));
#11404=CARTESIAN_POINT('Ctrl Pts',(2.8,57.3233277916702,2.00046370280581));
#11405=CARTESIAN_POINT('Ctrl Pts',(2.80651496136854,57.3688442456262,2.00740850907209));
#11406=CARTESIAN_POINT('Ctrl Pts',(2.83278587942622,57.4609346234663,2.03422841201581));
#11407=CARTESIAN_POINT('Ctrl Pts',(2.85367658846432,57.5051794406759,2.0551738220974));
#11408=CARTESIAN_POINT('Ctrl Pts',(2.91264660817257,57.5950293001724,2.11357045087714));
#11409=CARTESIAN_POINT('Ctrl Pts',(2.95372899720548,57.6363582268879,2.15381041488786));
#11410=CARTESIAN_POINT('Ctrl Pts',(3.04719526219676,57.7037440534718,2.24472494887073));
#11411=CARTESIAN_POINT('Ctrl Pts',(3.10085066357071,57.7281426935397,2.29658544858127));
#11412=CARTESIAN_POINT('Ctrl Pts',(3.21310392137581,57.7576460364624,2.40487775337108));
#11413=CARTESIAN_POINT('Ctrl Pts',(3.27253044418014,57.7618592555108,2.46210260432533));
#11414=CARTESIAN_POINT('Ctrl Pts',(3.33207315475466,57.7556502890388,2.51964428176073));
#11415=CARTESIAN_POINT('Ctrl Pts',(3.33316746036322,57.7555325268421,2.52070188444643));
#11416=CARTESIAN_POINT('Ctrl Pts',(3.33426151832784,57.7554111397819,2.5217593230988));
#11417=CARTESIAN_POINT('Ctrl Pts',(2.79999999999999,57.2767052616368,2.00002239837056));
#11418=CARTESIAN_POINT('Ctrl Pts',(2.79999999999999,57.2751280778309,2.00000746957523));
#11419=CARTESIAN_POINT('Ctrl Pts',(2.79999999999993,57.273550476778,2.));
#11420=CARTESIAN_POINT('Ctrl Pts',(2.79999999999993,57.2719725101481,2.));
#11421=CARTESIAN_POINT('Ctrl Pts',(7.6,51.,0.));
#11422=CARTESIAN_POINT('Ctrl Pts',(7.6,51.,51.));
#11423=CARTESIAN_POINT('Ctrl Pts',(7.6,0.,51.));
#11424=CARTESIAN_POINT('Ctrl Pts',(7.6,-51.,51.));
#11425=CARTESIAN_POINT('Ctrl Pts',(7.6,-51.,0.));
#11426=CARTESIAN_POINT('Ctrl Pts',(7.6,-51.,-51.));
#11427=CARTESIAN_POINT('Ctrl Pts',(7.6,0.,-51.));
#11428=CARTESIAN_POINT('Ctrl Pts',(7.6,51.,-51.));
#11429=CARTESIAN_POINT('Ctrl Pts',(7.6,51.,0.));
#11430=CARTESIAN_POINT('Ctrl Pts',(7.59004574184823,51.1988330750386,0.));
#11431=CARTESIAN_POINT('Ctrl Pts',(7.59004574184823,51.1988330750386,51.1988330750386));
#11432=CARTESIAN_POINT('Ctrl Pts',(7.59004574184823,0.,51.1988330750386));
#11433=CARTESIAN_POINT('Ctrl Pts',(7.59004574184823,-51.1988330750386,51.1988330750386));
#11434=CARTESIAN_POINT('Ctrl Pts',(7.59004574184823,-51.1988330750386,0.));
#11435=CARTESIAN_POINT('Ctrl Pts',(7.59004574184823,-51.1988330750386,-51.1988330750386));
#11436=CARTESIAN_POINT('Ctrl Pts',(7.59004574184823,0.,-51.1988330750386));
#11437=CARTESIAN_POINT('Ctrl Pts',(7.59004574184823,51.1988330750386,-51.1988330750386));
#11438=CARTESIAN_POINT('Ctrl Pts',(7.59004574184823,51.1988330750386,0.));
#11439=CARTESIAN_POINT('Ctrl Pts',(7.56669216920305,51.5895935047463,0.));
#11440=CARTESIAN_POINT('Ctrl Pts',(7.56669216920305,51.5895935047463,51.5895935047463));
#11441=CARTESIAN_POINT('Ctrl Pts',(7.56669216920305,0.,51.5895935047463));
#11442=CARTESIAN_POINT('Ctrl Pts',(7.56669216920305,-51.5895935047463,51.5895935047463));
#11443=CARTESIAN_POINT('Ctrl Pts',(7.56669216920305,-51.5895935047463,0.));
#11444=CARTESIAN_POINT('Ctrl Pts',(7.56669216920305,-51.5895935047463,-51.5895935047463));
#11445=CARTESIAN_POINT('Ctrl Pts',(7.56669216920305,0.,-51.5895935047463));
#11446=CARTESIAN_POINT('Ctrl Pts',(7.56669216920305,51.5895935047463,-51.5895935047463));
#11447=CARTESIAN_POINT('Ctrl Pts',(7.56669216920305,51.5895935047463,0.));
#11448=CARTESIAN_POINT('Ctrl Pts',(7.52132668197793,52.1550170184989,0.));
#11449=CARTESIAN_POINT('Ctrl Pts',(7.52132668197793,52.1550170184989,52.1550170184989));
#11450=CARTESIAN_POINT('Ctrl Pts',(7.52132668197793,0.,52.1550170184989));
#11451=CARTESIAN_POINT('Ctrl Pts',(7.52132668197793,-52.1550170184989,52.1550170184989));
#11452=CARTESIAN_POINT('Ctrl Pts',(7.52132668197793,-52.1550170184989,0.));
#11453=CARTESIAN_POINT('Ctrl Pts',(7.52132668197793,-52.1550170184989,-52.1550170184989));
#11454=CARTESIAN_POINT('Ctrl Pts',(7.52132668197793,0.,-52.1550170184989));
#11455=CARTESIAN_POINT('Ctrl Pts',(7.52132668197793,52.1550170184989,-52.1550170184989));
#11456=CARTESIAN_POINT('Ctrl Pts',(7.52132668197793,52.1550170184989,0.));
#11457=CARTESIAN_POINT('Ctrl Pts',(7.4400844252614,52.8673114594784,0.));
#11458=CARTESIAN_POINT('Ctrl Pts',(7.4400844252614,52.8673114594784,52.8673114594784));
#11459=CARTESIAN_POINT('Ctrl Pts',(7.4400844252614,0.,52.8673114594784));
#11460=CARTESIAN_POINT('Ctrl Pts',(7.4400844252614,-52.8673114594784,52.8673114594784));
#11461=CARTESIAN_POINT('Ctrl Pts',(7.4400844252614,-52.8673114594784,0.));
#11462=CARTESIAN_POINT('Ctrl Pts',(7.4400844252614,-52.8673114594784,-52.8673114594784));
#11463=CARTESIAN_POINT('Ctrl Pts',(7.4400844252614,0.,-52.8673114594784));
#11464=CARTESIAN_POINT('Ctrl Pts',(7.4400844252614,52.8673114594784,-52.8673114594784));
#11465=CARTESIAN_POINT('Ctrl Pts',(7.4400844252614,52.8673114594784,0.));
#11466=CARTESIAN_POINT('Ctrl Pts',(7.303261488895,53.6872261791492,0.));
#11467=CARTESIAN_POINT('Ctrl Pts',(7.303261488895,53.6872261791492,53.6872261791492));
#11468=CARTESIAN_POINT('Ctrl Pts',(7.303261488895,0.,53.6872261791492));
#11469=CARTESIAN_POINT('Ctrl Pts',(7.303261488895,-53.6872261791492,53.6872261791492));
#11470=CARTESIAN_POINT('Ctrl Pts',(7.303261488895,-53.6872261791492,0.));
#11471=CARTESIAN_POINT('Ctrl Pts',(7.303261488895,-53.6872261791492,-53.6872261791492));
#11472=CARTESIAN_POINT('Ctrl Pts',(7.303261488895,0.,-53.6872261791492));
#11473=CARTESIAN_POINT('Ctrl Pts',(7.303261488895,53.6872261791492,-53.6872261791492));
#11474=CARTESIAN_POINT('Ctrl Pts',(7.303261488895,53.6872261791492,0.));
#11475=CARTESIAN_POINT('Ctrl Pts',(7.1299954347016,54.4350859396526,0.));
#11476=CARTESIAN_POINT('Ctrl Pts',(7.1299954347016,54.4350859396526,54.4350859396526));
#11477=CARTESIAN_POINT('Ctrl Pts',(7.1299954347016,0.,54.4350859396526));
#11478=CARTESIAN_POINT('Ctrl Pts',(7.1299954347016,-54.4350859396526,54.4350859396526));
#11479=CARTESIAN_POINT('Ctrl Pts',(7.1299954347016,-54.4350859396526,0.));
#11480=CARTESIAN_POINT('Ctrl Pts',(7.1299954347016,-54.4350859396526,-54.4350859396526));
#11481=CARTESIAN_POINT('Ctrl Pts',(7.1299954347016,0.,-54.4350859396526));
#11482=CARTESIAN_POINT('Ctrl Pts',(7.1299954347016,54.4350859396526,-54.4350859396526));
#11483=CARTESIAN_POINT('Ctrl Pts',(7.1299954347016,54.4350859396526,0.));
#11484=CARTESIAN_POINT('Ctrl Pts',(6.91862269230318,55.1090497640848,0.));
#11485=CARTESIAN_POINT('Ctrl Pts',(6.91862269230318,55.1090497640848,55.1090497640848));
#11486=CARTESIAN_POINT('Ctrl Pts',(6.91862269230318,0.,55.1090497640848));
#11487=CARTESIAN_POINT('Ctrl Pts',(6.91862269230318,-55.1090497640848,55.1090497640848));
#11488=CARTESIAN_POINT('Ctrl Pts',(6.91862269230318,-55.1090497640848,0.));
#11489=CARTESIAN_POINT('Ctrl Pts',(6.91862269230318,-55.1090497640848,-55.1090497640848));
#11490=CARTESIAN_POINT('Ctrl Pts',(6.91862269230318,0.,-55.1090497640848));
#11491=CARTESIAN_POINT('Ctrl Pts',(6.91862269230318,55.1090497640848,-55.1090497640848));
#11492=CARTESIAN_POINT('Ctrl Pts',(6.91862269230318,55.1090497640848,0.));
#11493=CARTESIAN_POINT('Ctrl Pts',(6.66699410333038,55.7073490432259,0.));
#11494=CARTESIAN_POINT('Ctrl Pts',(6.66699410333038,55.7073490432258,55.7073490432258));
#11495=CARTESIAN_POINT('Ctrl Pts',(6.66699410333038,0.,55.7073490432259));
#11496=CARTESIAN_POINT('Ctrl Pts',(6.66699410333038,-55.7073490432258,55.7073490432258));
#11497=CARTESIAN_POINT('Ctrl Pts',(6.66699410333038,-55.7073490432259,0.));
#11498=CARTESIAN_POINT('Ctrl Pts',(6.66699410333038,-55.7073490432258,-55.7073490432258));
#11499=CARTESIAN_POINT('Ctrl Pts',(6.66699410333038,0.,-55.7073490432259));
#11500=CARTESIAN_POINT('Ctrl Pts',(6.66699410333038,55.7073490432258,-55.7073490432258));
#11501=CARTESIAN_POINT('Ctrl Pts',(6.66699410333038,55.7073490432259,0.));
#11502=CARTESIAN_POINT('Ctrl Pts',(6.37255361362915,56.2286342531435,0.));
#11503=CARTESIAN_POINT('Ctrl Pts',(6.37255361362915,56.2286342531435,56.2286342531435));
#11504=CARTESIAN_POINT('Ctrl Pts',(6.37255361362915,0.,56.2286342531435));
#11505=CARTESIAN_POINT('Ctrl Pts',(6.37255361362915,-56.2286342531435,56.2286342531435));
#11506=CARTESIAN_POINT('Ctrl Pts',(6.37255361362915,-56.2286342531435,0.));
#11507=CARTESIAN_POINT('Ctrl Pts',(6.37255361362915,-56.2286342531435,-56.2286342531435));
#11508=CARTESIAN_POINT('Ctrl Pts',(6.37255361362915,0.,-56.2286342531435));
#11509=CARTESIAN_POINT('Ctrl Pts',(6.37255361362915,56.2286342531435,-56.2286342531435));
#11510=CARTESIAN_POINT('Ctrl Pts',(6.37255361362915,56.2286342531435,0.));
#11511=CARTESIAN_POINT('Ctrl Pts',(6.03231545780073,56.6724462969604,0.));
#11512=CARTESIAN_POINT('Ctrl Pts',(6.03231545780073,56.6724462969604,56.6724462969604));
#11513=CARTESIAN_POINT('Ctrl Pts',(6.03231545780073,0.,56.6724462969604));
#11514=CARTESIAN_POINT('Ctrl Pts',(6.03231545780073,-56.6724462969604,56.6724462969604));
#11515=CARTESIAN_POINT('Ctrl Pts',(6.03231545780073,-56.6724462969604,0.));
#11516=CARTESIAN_POINT('Ctrl Pts',(6.03231545780073,-56.6724462969604,-56.6724462969604));
#11517=CARTESIAN_POINT('Ctrl Pts',(6.03231545780073,0.,-56.6724462969604));
#11518=CARTESIAN_POINT('Ctrl Pts',(6.03231545780073,56.6724462969604,-56.6724462969604));
#11519=CARTESIAN_POINT('Ctrl Pts',(6.03231545780073,56.6724462969604,0.));
#11520=CARTESIAN_POINT('Ctrl Pts',(5.64378712881462,57.0393576788909,0.));
#11521=CARTESIAN_POINT('Ctrl Pts',(5.64378712881462,57.0393576788909,57.0393576788909));
#11522=CARTESIAN_POINT('Ctrl Pts',(5.64378712881462,0.,57.0393576788909));
#11523=CARTESIAN_POINT('Ctrl Pts',(5.64378712881462,-57.0393576788909,57.0393576788909));
#11524=CARTESIAN_POINT('Ctrl Pts',(5.64378712881462,-57.0393576788909,0.));
#11525=CARTESIAN_POINT('Ctrl Pts',(5.64378712881462,-57.0393576788909,-57.0393576788909));
#11526=CARTESIAN_POINT('Ctrl Pts',(5.64378712881462,0.,-57.0393576788909));
#11527=CARTESIAN_POINT('Ctrl Pts',(5.64378712881462,57.0393576788909,-57.0393576788909));
#11528=CARTESIAN_POINT('Ctrl Pts',(5.64378712881462,57.0393576788909,0.));
#11529=CARTESIAN_POINT('Ctrl Pts',(5.20620249661537,57.331109156058,0.));
#11530=CARTESIAN_POINT('Ctrl Pts',(5.20620249661537,57.331109156058,57.331109156058));
#11531=CARTESIAN_POINT('Ctrl Pts',(5.20620249661537,0.,57.331109156058));
#11532=CARTESIAN_POINT('Ctrl Pts',(5.20620249661537,-57.331109156058,57.331109156058));
#11533=CARTESIAN_POINT('Ctrl Pts',(5.20620249661537,-57.331109156058,0.));
#11534=CARTESIAN_POINT('Ctrl Pts',(5.20620249661537,-57.331109156058,-57.331109156058));
#11535=CARTESIAN_POINT('Ctrl Pts',(5.20620249661537,0.,-57.331109156058));
#11536=CARTESIAN_POINT('Ctrl Pts',(5.20620249661537,57.331109156058,-57.331109156058));
#11537=CARTESIAN_POINT('Ctrl Pts',(5.20620249661537,57.331109156058,0.));
#11538=CARTESIAN_POINT('Ctrl Pts',(4.72163375439117,57.5508140869366,0.));
#11539=CARTESIAN_POINT('Ctrl Pts',(4.72163375439117,57.5508140869366,57.5508140869366));
#11540=CARTESIAN_POINT('Ctrl Pts',(4.72163375439117,0.,57.5508140869366));
#11541=CARTESIAN_POINT('Ctrl Pts',(4.72163375439117,-57.5508140869366,57.5508140869366));
#11542=CARTESIAN_POINT('Ctrl Pts',(4.72163375439117,-57.5508140869366,0.));
#11543=CARTESIAN_POINT('Ctrl Pts',(4.72163375439117,-57.5508140869366,-57.5508140869366));
#11544=CARTESIAN_POINT('Ctrl Pts',(4.72163375439117,0.,-57.5508140869366));
#11545=CARTESIAN_POINT('Ctrl Pts',(4.72163375439117,57.5508140869366,-57.5508140869366));
#11546=CARTESIAN_POINT('Ctrl Pts',(4.72163375439117,57.5508140869366,0.));
#11547=CARTESIAN_POINT('Ctrl Pts',(4.19645380044969,57.7033168044223,0.));
#11548=CARTESIAN_POINT('Ctrl Pts',(4.19645380044969,57.7033168044223,57.7033168044223));
#11549=CARTESIAN_POINT('Ctrl Pts',(4.19645380044969,0.,57.7033168044223));
#11550=CARTESIAN_POINT('Ctrl Pts',(4.19645380044969,-57.7033168044223,57.7033168044223));
#11551=CARTESIAN_POINT('Ctrl Pts',(4.19645380044969,-57.7033168044223,0.));
#11552=CARTESIAN_POINT('Ctrl Pts',(4.19645380044969,-57.7033168044223,-57.7033168044223));
#11553=CARTESIAN_POINT('Ctrl Pts',(4.19645380044969,0.,-57.7033168044223));
#11554=CARTESIAN_POINT('Ctrl Pts',(4.19645380044969,57.7033168044223,-57.7033168044223));
#11555=CARTESIAN_POINT('Ctrl Pts',(4.19645380044969,57.7033168044223,0.));
#11556=CARTESIAN_POINT('Ctrl Pts',(3.64216788966644,57.7953691453965,0.));
#11557=CARTESIAN_POINT('Ctrl Pts',(3.64216788966644,57.7953691453965,57.7953691453965));
#11558=CARTESIAN_POINT('Ctrl Pts',(3.64216788966644,0.,57.7953691453965));
#11559=CARTESIAN_POINT('Ctrl Pts',(3.64216788966644,-57.7953691453965,57.7953691453965));
#11560=CARTESIAN_POINT('Ctrl Pts',(3.64216788966644,-57.7953691453965,0.));
#11561=CARTESIAN_POINT('Ctrl Pts',(3.64216788966644,-57.7953691453965,-57.7953691453965));
#11562=CARTESIAN_POINT('Ctrl Pts',(3.64216788966644,0.,-57.7953691453965));
#11563=CARTESIAN_POINT('Ctrl Pts',(3.64216788966644,57.7953691453965,-57.7953691453965));
#11564=CARTESIAN_POINT('Ctrl Pts',(3.64216788966644,57.7953691453965,0.));
#11565=CARTESIAN_POINT('Ctrl Pts',(3.07295993429612,57.8346034867151,0.));
#11566=CARTESIAN_POINT('Ctrl Pts',(3.07295993429612,57.8346034867151,57.8346034867151));
#11567=CARTESIAN_POINT('Ctrl Pts',(3.07295993429612,0.,57.8346034867151));
#11568=CARTESIAN_POINT('Ctrl Pts',(3.07295993429612,-57.8346034867151,57.8346034867151));
#11569=CARTESIAN_POINT('Ctrl Pts',(3.07295993429612,-57.8346034867151,0.));
#11570=CARTESIAN_POINT('Ctrl Pts',(3.07295993429612,-57.8346034867151,-57.8346034867151));
#11571=CARTESIAN_POINT('Ctrl Pts',(3.07295993429612,0.,-57.8346034867151));
#11572=CARTESIAN_POINT('Ctrl Pts',(3.07295993429612,57.8346034867151,-57.8346034867151));
#11573=CARTESIAN_POINT('Ctrl Pts',(3.07295993429612,57.8346034867151,0.));
#11574=CARTESIAN_POINT('Ctrl Pts',(2.50364225081115,57.8287013224614,0.));
#11575=CARTESIAN_POINT('Ctrl Pts',(2.50364225081115,57.8287013224614,57.8287013224614));
#11576=CARTESIAN_POINT('Ctrl Pts',(2.50364225081115,0.,57.8287013224614));
#11577=CARTESIAN_POINT('Ctrl Pts',(2.50364225081115,-57.8287013224614,57.8287013224614));
#11578=CARTESIAN_POINT('Ctrl Pts',(2.50364225081115,-57.8287013224614,0.));
#11579=CARTESIAN_POINT('Ctrl Pts',(2.50364225081115,-57.8287013224614,-57.8287013224614));
#11580=CARTESIAN_POINT('Ctrl Pts',(2.50364225081115,0.,-57.8287013224614));
#11581=CARTESIAN_POINT('Ctrl Pts',(2.50364225081115,57.8287013224614,-57.8287013224614));
#11582=CARTESIAN_POINT('Ctrl Pts',(2.50364225081115,57.8287013224614,0.));
#11583=CARTESIAN_POINT('Ctrl Pts',(1.94767564770796,57.7846117731639,0.));
#11584=CARTESIAN_POINT('Ctrl Pts',(1.94767564770796,57.7846117731638,57.7846117731638));
#11585=CARTESIAN_POINT('Ctrl Pts',(1.94767564770796,0.,57.7846117731639));
#11586=CARTESIAN_POINT('Ctrl Pts',(1.94767564770796,-57.7846117731638,57.7846117731638));
#11587=CARTESIAN_POINT('Ctrl Pts',(1.94767564770796,-57.7846117731639,0.));
#11588=CARTESIAN_POINT('Ctrl Pts',(1.94767564770796,-57.7846117731638,-57.7846117731638));
#11589=CARTESIAN_POINT('Ctrl Pts',(1.94767564770796,0.,-57.7846117731639));
#11590=CARTESIAN_POINT('Ctrl Pts',(1.94767564770796,57.7846117731638,-57.7846117731638));
#11591=CARTESIAN_POINT('Ctrl Pts',(1.94767564770796,57.7846117731639,0.));
#11592=CARTESIAN_POINT('Ctrl Pts',(1.41470323398176,57.7076450358389,0.));
#11593=CARTESIAN_POINT('Ctrl Pts',(1.41470323398176,57.7076450358389,57.7076450358389));
#11594=CARTESIAN_POINT('Ctrl Pts',(1.41470323398176,0.,57.7076450358389));
#11595=CARTESIAN_POINT('Ctrl Pts',(1.41470323398176,-57.7076450358389,57.7076450358389));
#11596=CARTESIAN_POINT('Ctrl Pts',(1.41470323398176,-57.7076450358389,0.));
#11597=CARTESIAN_POINT('Ctrl Pts',(1.41470323398176,-57.7076450358389,-57.7076450358389));
#11598=CARTESIAN_POINT('Ctrl Pts',(1.41470323398176,0.,-57.7076450358389));
#11599=CARTESIAN_POINT('Ctrl Pts',(1.41470323398176,57.7076450358389,-57.7076450358389));
#11600=CARTESIAN_POINT('Ctrl Pts',(1.41470323398176,57.7076450358389,0.));
#11601=CARTESIAN_POINT('Ctrl Pts',(0.909896369306813,57.6011916129045,0.));
#11602=CARTESIAN_POINT('Ctrl Pts',(0.909896369306813,57.6011916129045,57.6011916129045));
#11603=CARTESIAN_POINT('Ctrl Pts',(0.909896369306813,0.,57.6011916129045));
#11604=CARTESIAN_POINT('Ctrl Pts',(0.909896369306813,-57.6011916129045,
57.6011916129045));
#11605=CARTESIAN_POINT('Ctrl Pts',(0.909896369306813,-57.6011916129045,
0.));
#11606=CARTESIAN_POINT('Ctrl Pts',(0.909896369306813,-57.6011916129045,
-57.6011916129045));
#11607=CARTESIAN_POINT('Ctrl Pts',(0.909896369306813,0.,-57.6011916129045));
#11608=CARTESIAN_POINT('Ctrl Pts',(0.909896369306813,57.6011916129045,-57.6011916129045));
#11609=CARTESIAN_POINT('Ctrl Pts',(0.909896369306813,57.6011916129045,0.));
#11610=CARTESIAN_POINT('Ctrl Pts',(0.530456882251734,57.4940201174365,0.));
#11611=CARTESIAN_POINT('Ctrl Pts',(0.530456882251734,57.4940201174365,57.4940201174365));
#11612=CARTESIAN_POINT('Ctrl Pts',(0.530456882251733,0.,57.4940201174365));
#11613=CARTESIAN_POINT('Ctrl Pts',(0.530456882251732,-57.4940201174365,
57.4940201174365));
#11614=CARTESIAN_POINT('Ctrl Pts',(0.530456882251732,-57.4940201174365,
0.));
#11615=CARTESIAN_POINT('Ctrl Pts',(0.530456882251732,-57.4940201174365,
-57.4940201174365));
#11616=CARTESIAN_POINT('Ctrl Pts',(0.530456882251733,0.,-57.4940201174365));
#11617=CARTESIAN_POINT('Ctrl Pts',(0.530456882251734,57.4940201174365,-57.4940201174365));
#11618=CARTESIAN_POINT('Ctrl Pts',(0.530456882251734,57.4940201174365,0.));
#11619=CARTESIAN_POINT('Ctrl Pts',(0.25982504671998,57.4016528748871,0.));
#11620=CARTESIAN_POINT('Ctrl Pts',(0.25982504671998,57.4016528748871,57.4016528748871));
#11621=CARTESIAN_POINT('Ctrl Pts',(0.259825046719979,0.,57.4016528748871));
#11622=CARTESIAN_POINT('Ctrl Pts',(0.259825046719979,-57.4016528748871,
57.4016528748871));
#11623=CARTESIAN_POINT('Ctrl Pts',(0.259825046719979,-57.4016528748871,
0.));
#11624=CARTESIAN_POINT('Ctrl Pts',(0.259825046719979,-57.4016528748871,
-57.4016528748871));
#11625=CARTESIAN_POINT('Ctrl Pts',(0.259825046719979,0.,-57.4016528748871));
#11626=CARTESIAN_POINT('Ctrl Pts',(0.25982504671998,57.4016528748871,-57.4016528748871));
#11627=CARTESIAN_POINT('Ctrl Pts',(0.25982504671998,57.4016528748871,0.));
#11628=CARTESIAN_POINT('Ctrl Pts',(0.0855791821307019,57.3347686565506,
0.));
#11629=CARTESIAN_POINT('Ctrl Pts',(0.0855791821307019,57.3347686565505,
57.3347686565505));
#11630=CARTESIAN_POINT('Ctrl Pts',(0.0855791821307017,0.,57.3347686565506));
#11631=CARTESIAN_POINT('Ctrl Pts',(0.0855791821307015,-57.3347686565505,
57.3347686565505));
#11632=CARTESIAN_POINT('Ctrl Pts',(0.0855791821307015,-57.3347686565506,
0.));
#11633=CARTESIAN_POINT('Ctrl Pts',(0.0855791821307015,-57.3347686565505,
-57.3347686565505));
#11634=CARTESIAN_POINT('Ctrl Pts',(0.0855791821307017,0.,-57.3347686565506));
#11635=CARTESIAN_POINT('Ctrl Pts',(0.0855791821307019,57.3347686565505,
-57.3347686565505));
#11636=CARTESIAN_POINT('Ctrl Pts',(0.0855791821307019,57.3347686565506,
0.));
#11637=CARTESIAN_POINT('Ctrl Pts',(0.,57.3,0.));
#11638=CARTESIAN_POINT('Ctrl Pts',(0.,57.3,57.3));
#11639=CARTESIAN_POINT('Ctrl Pts',(0.,0.,57.3));
#11640=CARTESIAN_POINT('Ctrl Pts',(0.,-57.3,57.3));
#11641=CARTESIAN_POINT('Ctrl Pts',(0.,-57.3,0.));
#11642=CARTESIAN_POINT('Ctrl Pts',(0.,-57.3,-57.3));
#11643=CARTESIAN_POINT('Ctrl Pts',(0.,0.,-57.3));
#11644=CARTESIAN_POINT('Ctrl Pts',(0.,57.3,-57.3));
#11645=CARTESIAN_POINT('Ctrl Pts',(0.,57.3,0.));
#11646=CARTESIAN_POINT('',(3.33426151832784,57.7554111397819,-2.5217593230988));
#11647=CARTESIAN_POINT('Ctrl Pts',(3.33426151832794,57.7554111397819,-2.5217593230988));
#11648=CARTESIAN_POINT('Ctrl Pts',(2.31390369740531,57.8158698649553,-2.52187727319098));
#11649=CARTESIAN_POINT('Ctrl Pts',(1.31472805667171,57.6929865211876,-2.52171535509756));
#11650=CARTESIAN_POINT('Ctrl Pts',(0.339274733856492,57.3708526295189,-2.52078316017081));
#11651=CARTESIAN_POINT('',(3.33426151832786,57.8104383827772,4.21884749357559E-14));
#11652=CARTESIAN_POINT('Ctrl Pts',(3.33426151832784,57.8104299775689,8.7513329916078E-12));
#11653=CARTESIAN_POINT('Ctrl Pts',(3.33426151832784,57.8104299773062,-0.840857117582111));
#11654=CARTESIAN_POINT('Ctrl Pts',(3.33426151832784,57.792090085957,-1.68170785699931));
#11655=CARTESIAN_POINT('Ctrl Pts',(3.33426151832784,57.7554111397819,-2.5217593230989));
#11656=CARTESIAN_POINT('Ctrl Pts',(3.33426151832786,57.8104383827772,0.));
#11657=CARTESIAN_POINT('Ctrl Pts',(3.39537650339183,57.8062407319816,0.));
#11658=CARTESIAN_POINT('Ctrl Pts',(3.56948527592296,57.7922402732231,0.));
#11659=CARTESIAN_POINT('Ctrl Pts',(3.85481788311223,57.7593613281302,0.));
#11660=CARTESIAN_POINT('Ctrl Pts',(4.24482380713023,57.6892710332381,0.));
#11661=CARTESIAN_POINT('Ctrl Pts',(4.72163375439117,57.5508140869366,0.));
#11662=CARTESIAN_POINT('Ctrl Pts',(5.20620249661537,57.331109156058,0.));
#11663=CARTESIAN_POINT('Ctrl Pts',(5.64378712881462,57.0393576788909,0.));
#11664=CARTESIAN_POINT('Ctrl Pts',(6.03231545780073,56.6724462969604,0.));
#11665=CARTESIAN_POINT('Ctrl Pts',(6.37255361362915,56.2286342531435,0.));
#11666=CARTESIAN_POINT('Ctrl Pts',(6.66699410333038,55.7073490432259,0.));
#11667=CARTESIAN_POINT('Ctrl Pts',(6.91862269230318,55.1090497640848,0.));
#11668=CARTESIAN_POINT('Ctrl Pts',(7.1299954347016,54.4350859396526,0.));
#11669=CARTESIAN_POINT('Ctrl Pts',(7.303261488895,53.6872261791492,0.));
#11670=CARTESIAN_POINT('Ctrl Pts',(7.4400844252614,52.8673114594784,0.));
#11671=CARTESIAN_POINT('Ctrl Pts',(7.52132668197793,52.1550170184989,0.));
#11672=CARTESIAN_POINT('Ctrl Pts',(7.56669216920305,51.5895935047463,0.));
#11673=CARTESIAN_POINT('Ctrl Pts',(7.59004574184823,51.1988330750386,0.));
#11674=CARTESIAN_POINT('Ctrl Pts',(7.6,51.,0.));
#11675=CARTESIAN_POINT('Ctrl Pts',(3.33426151832784,57.7554111397819,2.5217593230988));
#11676=CARTESIAN_POINT('Ctrl Pts',(3.33426151832784,57.7920906439767,1.68169507677206));
#11677=CARTESIAN_POINT('Ctrl Pts',(3.33426151832784,57.8104299778316,0.840844349400496));
#11678=CARTESIAN_POINT('Ctrl Pts',(3.33426151832784,57.8104299775689,8.89477380638937E-12));
#11679=CARTESIAN_POINT('Ctrl Pts',(0.499999999999865,56.8978458123625,-2.));
#11680=CARTESIAN_POINT('Ctrl Pts',(1.39877068709361,57.1962523550952,-2.));
#11681=CARTESIAN_POINT('Ctrl Pts',(2.35587473833157,57.3142929108325,-2.));
#11682=CARTESIAN_POINT('Ctrl Pts',(3.30000000000009,57.2570611822017,-2.));
#11683=CARTESIAN_POINT('Ctrl Pts',(0.411584403188717,57.1580487103768,-1.99244885315961));
#11684=CARTESIAN_POINT('Ctrl Pts',(1.3524312707013,57.4698597329914,-1.99241931647723));
#11685=CARTESIAN_POINT('Ctrl Pts',(2.33276518160068,57.5906485008099,-1.99241414329164));
#11686=CARTESIAN_POINT('Ctrl Pts',(3.318873716526,57.5315882986027,-1.99241789689239));
#11687=CARTESIAN_POINT('Ctrl Pts',(0.333172302665028,57.3888117943974,-2.24652030369265));
#11688=CARTESIAN_POINT('Ctrl Pts',(1.31137387294133,57.7123824082932,-2.24714501562381));
#11689=CARTESIAN_POINT('Ctrl Pts',(2.31227799847626,57.8355775691272,-2.24725411917667));
#11690=CARTESIAN_POINT('Ctrl Pts',(3.33560242564904,57.7749152697564,-2.24717484796589));
#11691=CARTESIAN_POINT('Ctrl Pts',(0.339274733856492,57.3708526295189,-2.52078316017081));
#11692=CARTESIAN_POINT('Ctrl Pts',(1.31472805667171,57.6929865211876,-2.52171535509756));
#11693=CARTESIAN_POINT('Ctrl Pts',(2.31390369740531,57.8158698649553,-2.52187727319098));
#11694=CARTESIAN_POINT('Ctrl Pts',(3.33426151832794,57.7554111397819,-2.5217593230988));
#11695=CARTESIAN_POINT('',(2.80000000000039,57.2719725101482,-2.));
#11696=CARTESIAN_POINT('Ctrl Pts',(0.499999999999865,56.8978458123625,-2.));
#11697=CARTESIAN_POINT('Ctrl Pts',(1.24037244163541,57.1436615513665,-2.));
#11698=CARTESIAN_POINT('Ctrl Pts',(2.02032888654137,57.267084078118,-2.));
#11699=CARTESIAN_POINT('Ctrl Pts',(2.80000655418616,57.2709607214293,-2.));
#11700=CARTESIAN_POINT('',(2.8,57.2767052616367,-2.00002239837057));
#11701=CARTESIAN_POINT('Ctrl Pts',(2.8,57.2719725101481,-2.));
#11702=CARTESIAN_POINT('Ctrl Pts',(2.8,57.2735503201058,-2.));
#11703=CARTESIAN_POINT('Ctrl Pts',(2.8,57.2751279214594,-2.0000074680951));
#11704=CARTESIAN_POINT('Ctrl Pts',(2.8,57.2767052616367,-2.00002239837056));
#11705=CARTESIAN_POINT('Ctrl Pts',(2.8,57.2767052616367,-2.00002239837056));
#11706=CARTESIAN_POINT('Ctrl Pts',(2.8,57.3233277916701,-2.0004637028058));
#11707=CARTESIAN_POINT('Ctrl Pts',(2.80651496136847,57.3688442456259,-2.00740850907196));
#11708=CARTESIAN_POINT('Ctrl Pts',(2.83278587942598,57.4609346234655,-2.03422841201549));
#11709=CARTESIAN_POINT('Ctrl Pts',(2.85367658846371,57.5051794406747,-2.05517382209671));
#11710=CARTESIAN_POINT('Ctrl Pts',(2.91264660817062,57.5950293001698,-2.11357045087513));
#11711=CARTESIAN_POINT('Ctrl Pts',(2.95372899720229,57.6363582268848,-2.15381041488474));
#11712=CARTESIAN_POINT('Ctrl Pts',(3.04719526219418,57.7037440534708,-2.24472494886825));
#11713=CARTESIAN_POINT('Ctrl Pts',(3.10085066357087,57.7281426935401,-2.29658544858143));
#11714=CARTESIAN_POINT('Ctrl Pts',(3.21310392137964,57.757646036463,-2.40487775337478));
#11715=CARTESIAN_POINT('Ctrl Pts',(3.27253044416714,57.7618592555105,-2.46210260436637));
#11716=CARTESIAN_POINT('Ctrl Pts',(3.33207315476026,57.7556502890384,-2.51964428176192));
#11717=CARTESIAN_POINT('Ctrl Pts',(3.33316746036413,57.755532526842,-2.52070188444734));
#11718=CARTESIAN_POINT('Ctrl Pts',(3.33426151832784,57.7554111397819,-2.52175932309883));
#11719=CARTESIAN_POINT('Origin',(1.15,56.75,-2.));
#11720=CARTESIAN_POINT('',(2.8,55.,-2.));
#11721=CARTESIAN_POINT('Ctrl Pts',(2.8,55.3431808226538,2.5000000000072));
#11722=CARTESIAN_POINT('Ctrl Pts',(2.8,55.418416750227,0.834481782395201));
#11723=CARTESIAN_POINT('Ctrl Pts',(2.8,55.4184191500722,-0.834428656364044));
#11724=CARTESIAN_POINT('Ctrl Pts',(2.8,55.3431808226542,-2.50000000000005));
#11725=CARTESIAN_POINT('Ctrl Pts',(2.8,55.2009701963905,2.493575964374));
#11726=CARTESIAN_POINT('Ctrl Pts',(2.8,55.2760124216453,0.832345787733798));
#11727=CARTESIAN_POINT('Ctrl Pts',(2.8,55.2760148153119,-0.832292798480848));
#11728=CARTESIAN_POINT('Ctrl Pts',(2.8,55.2009701963908,-2.49357596436687));
#11729=CARTESIAN_POINT('Ctrl Pts',(2.86422761419582,55.0599778981397,2.4872069638867));
#11730=CARTESIAN_POINT('Ctrl Pts',(2.86422761419582,55.1348283214914,0.830222758207451));
#11731=CARTESIAN_POINT('Ctrl Pts',(2.86422761419583,55.13483070904,-0.830169904390779));
#11732=CARTESIAN_POINT('Ctrl Pts',(2.86422761419583,55.05997789814,-2.48720696387959));
#11733=CARTESIAN_POINT('Ctrl Pts',(2.97156409628599,54.9665637470306,2.48298719598933));
#11734=CARTESIAN_POINT('Ctrl Pts',(2.97156409628599,55.0412876849674,0.828803032387072));
#11735=CARTESIAN_POINT('Ctrl Pts',(2.971564096286,55.0412900684814,-0.828750267885016));
#11736=CARTESIAN_POINT('Ctrl Pts',(2.971564096286,54.9665637470309,-2.48298719598223));
#11737=CARTESIAN_POINT('',(2.8,55.363504798459,2.00000000000001));
#11738=CARTESIAN_POINT('Ctrl Pts',(2.8,55.3599937696469,2.09491350990412));
#11739=CARTESIAN_POINT('Ctrl Pts',(2.8,55.3611908435143,2.06327665921582));
#11740=CARTESIAN_POINT('Ctrl Pts',(2.8,55.3623607880677,2.03163878205578));
#11741=CARTESIAN_POINT('Ctrl Pts',(2.8,55.3635036032579,1.99999992451711));
#11742=CARTESIAN_POINT('',(2.8,55.363504798459,-1.99999999999998));
#11743=CARTESIAN_POINT('Ctrl Pts',(2.8,55.3635036032579,1.99999992451718));
#11744=CARTESIAN_POINT('Ctrl Pts',(2.8,55.4116430788051,0.667257743744672));
#11745=CARTESIAN_POINT('Ctrl Pts',(2.8,55.4116443040882,-0.66722401754958));
#11746=CARTESIAN_POINT('Ctrl Pts',(2.8,55.363503594285,-2.00000017815421));
#11747=CARTESIAN_POINT('Ctrl Pts',(2.8,55.3599937633195,-2.0949136807012));
#11748=CARTESIAN_POINT('Ctrl Pts',(2.8,55.3611908369837,-2.06327683842182));
#11749=CARTESIAN_POINT('Ctrl Pts',(2.8,55.3623607806224,-2.03163898887636));
#11750=CARTESIAN_POINT('Ctrl Pts',(2.8,55.363503594285,-2.00000017815421));
#11751=CARTESIAN_POINT('Origin',(2.8,55.,0.));
#11752=CARTESIAN_POINT('',(2.8,57.2767060437521,1.99999999999997));
#11753=CARTESIAN_POINT('Ctrl Pts',(2.8,57.2767049572205,2.00000016086605));
#11754=CARTESIAN_POINT('Ctrl Pts',(2.8,57.2767046965456,2.00000762698538));
#11755=CARTESIAN_POINT('Ctrl Pts',(2.8,57.2767044358693,2.00001509310466));
#11756=CARTESIAN_POINT('Ctrl Pts',(2.8,57.2767041751915,2.0000225592239));
#11757=CARTESIAN_POINT('',(2.8,57.2767060437521,-1.99999999999999));
#11758=CARTESIAN_POINT('Ctrl Pts',(2.8,57.2767049649653,-1.99999993439379));
#11759=CARTESIAN_POINT('Ctrl Pts',(2.8,57.3232381590415,-0.667219180437501));
#11760=CARTESIAN_POINT('Ctrl Pts',(2.8,57.3232392879721,0.667187020901882));
#11761=CARTESIAN_POINT('Ctrl Pts',(2.8,57.2767049572205,2.00000016086605));
#11762=CARTESIAN_POINT('Ctrl Pts',(2.8,57.2767049649653,-1.99999993439379));
#11763=CARTESIAN_POINT('Ctrl Pts',(2.8,57.2767047042902,-2.00000740051943));
#11764=CARTESIAN_POINT('Ctrl Pts',(2.8,57.2767044436137,-2.00001486664502));
#11765=CARTESIAN_POINT('Ctrl Pts',(2.8,57.2767041829358,-2.00002233277056));
#11766=CARTESIAN_POINT('Ctrl Pts',(2.8,57.2570611822017,-2.50000000000011));
#11767=CARTESIAN_POINT('Ctrl Pts',(2.8,57.3297855444336,-0.834406696899876));
#11768=CARTESIAN_POINT('Ctrl Pts',(2.8,57.3297877551691,0.834356064814358));
#11769=CARTESIAN_POINT('Ctrl Pts',(2.8,57.2570611822017,2.50000000000002));
#11770=CARTESIAN_POINT('Ctrl Pts',(2.8,57.3935455699524,-2.50595928191804));
#11771=CARTESIAN_POINT('Ctrl Pts',(2.8,57.4664436708706,-0.836386872181238));
#11772=CARTESIAN_POINT('Ctrl Pts',(2.8,57.4664458868875,0.836336119135542));
#11773=CARTESIAN_POINT('Ctrl Pts',(2.8,57.3935455699524,2.50595928191794));
#11774=CARTESIAN_POINT('Ctrl Pts',(2.91867325002229,57.6650888139175,-2.51781560314543));
#11775=CARTESIAN_POINT('Ctrl Pts',(2.91867325002229,57.7383307514702,-0.840368363322168));
#11776=CARTESIAN_POINT('Ctrl Pts',(2.91867325002229,57.7383329779393,0.840317370890855));
#11777=CARTESIAN_POINT('Ctrl Pts',(2.91867325002229,57.6650888139175,2.51781560314534));
#11778=CARTESIAN_POINT('Ctrl Pts',(3.19796820075467,57.7647634644866,-2.5221676711922));
#11779=CARTESIAN_POINT('Ctrl Pts',(3.19796820075467,57.838134288488,-0.841768567659979));
#11780=CARTESIAN_POINT('Ctrl Pts',(3.19796820075467,57.8381365188751,0.841717485495471));
#11781=CARTESIAN_POINT('Ctrl Pts',(3.19796820075467,57.7647634644867,2.52216767119211));
#11782=CARTESIAN_POINT('Ctrl Pts',(3.33426151832784,57.7554111397819,-2.5217593230989));
#11783=CARTESIAN_POINT('Ctrl Pts',(3.33426151832784,57.8287684751718,-0.841669146865329));
#11784=CARTESIAN_POINT('Ctrl Pts',(3.33426151832784,57.8287707051489,0.841618074091848));
#11785=CARTESIAN_POINT('Ctrl Pts',(3.33426151832784,57.7554111397819,2.5217593230988));
#11786=CARTESIAN_POINT('Origin',(11.,20.,0.));
#11787=CARTESIAN_POINT('Origin',(0.3,0.,0.));
#12794=UNCERTAINTY_MEASURE_WITH_UNIT(LENGTH_MEASURE(0.01),#12814,
'DISTANCE_ACCURACY_VALUE',
'Maximum model space distance between geometric entities at asserted c
onnectivities');
#12801=UNCERTAINTY_MEASURE_WITH_UNIT(LENGTH_MEASURE(0.01),#12814,
'DISTANCE_ACCURACY_VALUE',
'Maximum model space distance between geometric entities at asserted c
onnectivities');
#12806=(
GEOMETRIC_REPRESENTATION_CONTEXT(3)
GLOBAL_UNCERTAINTY_ASSIGNED_CONTEXT((#12794))
GLOBAL_UNIT_ASSIGNED_CONTEXT((#12814,#12816,#12817))
REPRESENTATION_CONTEXT('','3D')
);
#12813=(
GEOMETRIC_REPRESENTATION_CONTEXT(3)
GLOBAL_UNCERTAINTY_ASSIGNED_CONTEXT((#12801))
GLOBAL_UNIT_ASSIGNED_CONTEXT((#12814,#12816,#12817))
REPRESENTATION_CONTEXT('','3D')
);
#12814=(
LENGTH_UNIT()
NAMED_UNIT(*)
SI_UNIT(.MILLI.,.METRE.)
);
#12816=(
NAMED_UNIT(*)
PLANE_ANGLE_UNIT()
SI_UNIT($,.RADIAN.)
);
#12817=(
NAMED_UNIT(*)
SI_UNIT($,.STERADIAN.)
SOLID_ANGLE_UNIT()
);
#12822=SHAPE_DEFINITION_REPRESENTATION(#12833,#12857);
#12833=PRODUCT_DEFINITION_SHAPE('',$,#12869);
#12857=SHAPE_REPRESENTATION('',(#4704),#12806);
#12864=PRODUCT_DEFINITION_CONTEXT('part definition',#12899,'design');
#12869=PRODUCT_DEFINITION('2026-10-11-12-17-35-580',
'04_Lower_Fixed_Sheave_Dish',#12880,#12864);
#12880=PRODUCT_DEFINITION_FORMATION('',$,#12905);
#12899=APPLICATION_CONTEXT(
'Core Data for Automotive Mechanical Design Process');
#12900=PRODUCT_CONTEXT('part definition',#12899,'mechanical');
#12905=PRODUCT('2026-10-11-12-17-35-580','04_Lower_Fixed_Sheave_Dish',$,
(#12900));
#12961=COLOUR_RGB('Sky Blue',0.24,0.69,0.87);
#12962=FILL_AREA_STYLE_COLOUR('',#12961);
#12963=FILL_AREA_STYLE('',(#12962));
#12964=SURFACE_STYLE_FILL_AREA(#12963);
#12965=SURFACE_SIDE_STYLE('',(#12964));
#12966=SURFACE_STYLE_USAGE(.BOTH.,#12965);
#12967=PRESENTATION_STYLE_ASSIGNMENT((#12966));
ENDSEC;
END-ISO-10303-21;
